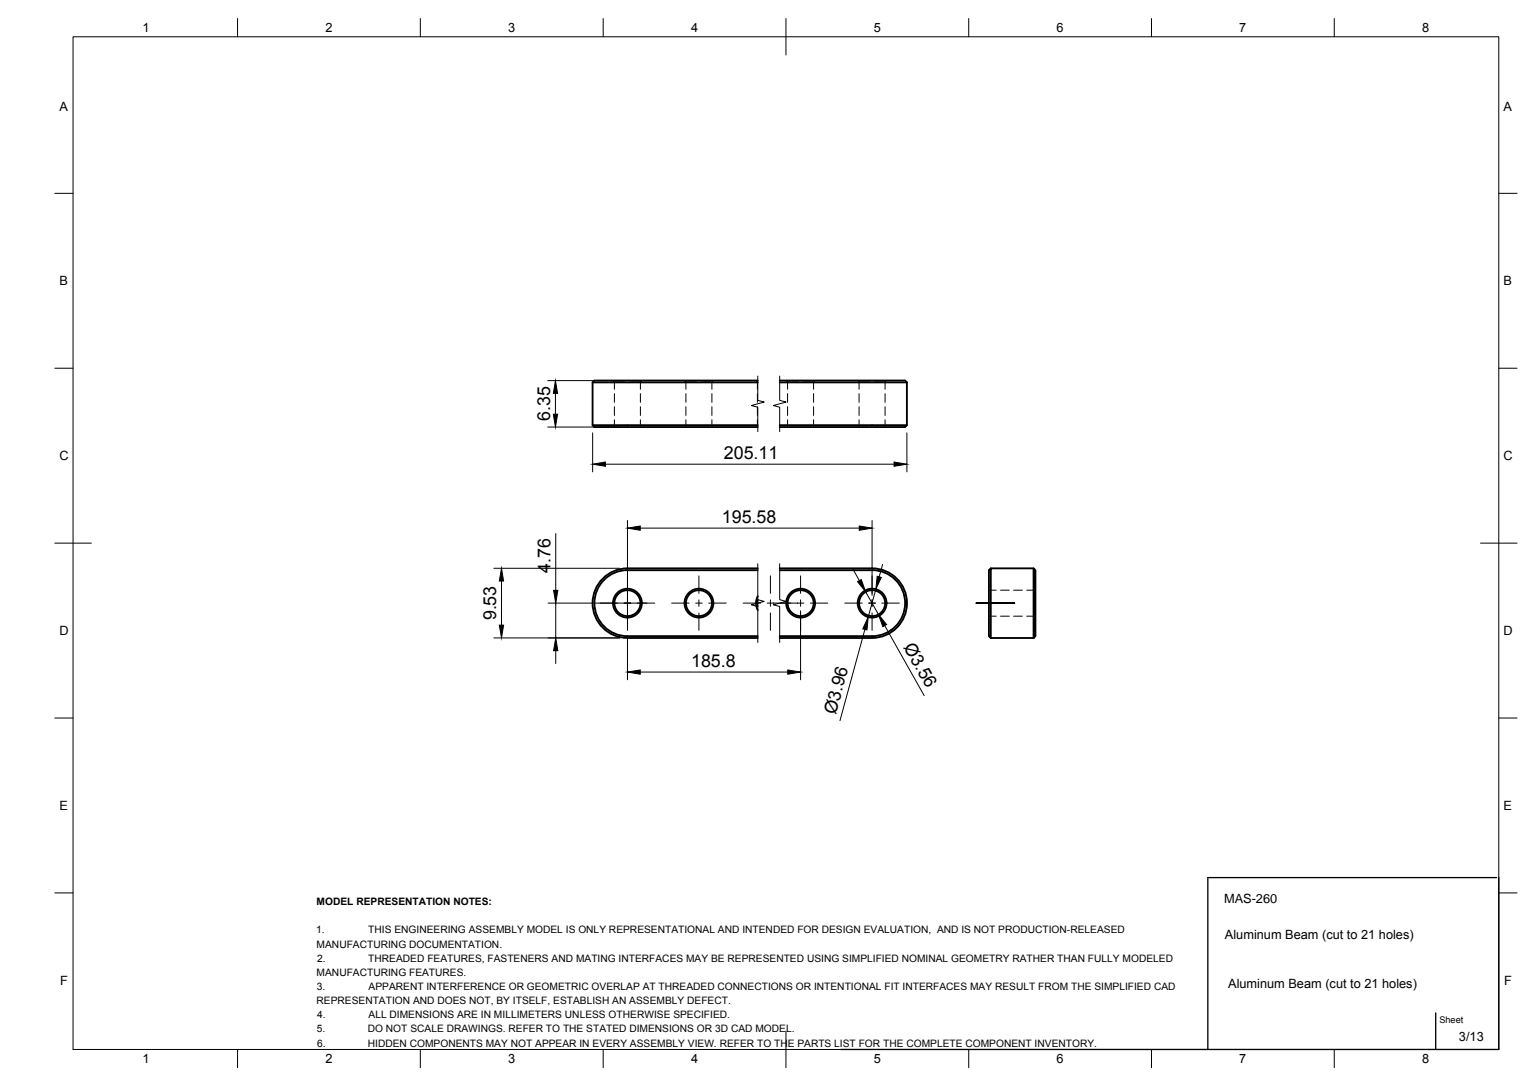
ISO-10303-21;
HEADER;
/* Generated by software containing ST-Developer
 * from STEP Tools, Inc. (www.steptools.com) 
 */

FILE_DESCRIPTION(
/* description */ (''),
/* implementation_level */ '2;1');

FILE_NAME(
/* name */ 'Aluminum Beam (cut to 21 holes).step',
/* time_stamp */ '2026-10-15T13:29:10-07:00',
/* author */ (''),
/* organization */ (''),
/* preprocessor_version */ 'ST-DEVELOPER v20.2',
/* originating_system */ 'Autodesk Translation Framework v15.15.0.0',
/* authorisation */ '');

FILE_SCHEMA (('AUTOMOTIVE_DESIGN { 1 0 10303 214 3 1 1 }'));
ENDSEC;

DATA;
#10=MECHANICAL_DESIGN_GEOMETRIC_PRESENTATION_REPRESENTATION('',(#938),#83219);
#910=SHAPE_REPRESENTATION_RELATIONSHIP('SRR','None',#83305,#924);
#924=ADVANCED_BREP_SHAPE_REPRESENTATION('',(#952),#83210);
#938=STYLED_ITEM('',(#83384),#952);
#952=MANIFOLD_SOLID_BREP('Body1',#26934);
#1019=FACE_BOUND('',#4280,.T.);
#1020=FACE_BOUND('',#4281,.T.);
#1021=FACE_BOUND('',#4282,.T.);
#1022=FACE_BOUND('',#4283,.T.);
#1023=FACE_BOUND('',#4284,.T.);
#1024=FACE_BOUND('',#4285,.T.);
#1025=FACE_BOUND('',#4286,.T.);
#1026=FACE_BOUND('',#4287,.T.);
#1027=FACE_BOUND('',#4288,.T.);
#1028=FACE_BOUND('',#4289,.T.);
#1029=FACE_BOUND('',#4290,.T.);
#1030=FACE_BOUND('',#4291,.T.);
#1031=FACE_BOUND('',#4292,.T.);
#1032=FACE_BOUND('',#4293,.T.);
#1033=FACE_BOUND('',#4294,.T.);
#1034=FACE_BOUND('',#4295,.T.);
#1035=FACE_BOUND('',#4296,.T.);
#1036=FACE_BOUND('',#4297,.T.);
#1037=FACE_BOUND('',#4298,.T.);
#1038=FACE_BOUND('',#4299,.T.);
#1039=FACE_BOUND('',#4300,.T.);
#1040=FACE_BOUND('',#4354,.T.);
#1041=FACE_BOUND('',#4355,.T.);
#1042=FACE_BOUND('',#4356,.T.);
#1043=FACE_BOUND('',#4357,.T.);
#1044=FACE_BOUND('',#4358,.T.);
#1045=FACE_BOUND('',#4359,.T.);
#1046=FACE_BOUND('',#4360,.T.);
#1047=FACE_BOUND('',#4361,.T.);
#1048=FACE_BOUND('',#4362,.T.);
#1049=FACE_BOUND('',#4363,.T.);
#1050=FACE_BOUND('',#4364,.T.);
#1051=FACE_BOUND('',#4365,.T.);
#1052=FACE_BOUND('',#4366,.T.);
#1053=FACE_BOUND('',#4367,.T.);
#1054=FACE_BOUND('',#4368,.T.);
#1055=FACE_BOUND('',#4369,.T.);
#1056=FACE_BOUND('',#4370,.T.);
#1057=FACE_BOUND('',#4371,.T.);
#1058=FACE_BOUND('',#4372,.T.);
#1059=FACE_BOUND('',#4373,.T.);
#1060=FACE_BOUND('',#4374,.T.);
#1415=PLANE('',#27876);
#1416=PLANE('',#27981);
#1417=PLANE('',#27984);
#1418=PLANE('',#27989);
#1419=PLANE('',#27990);
#1420=PLANE('',#27994);
#1421=PLANE('',#27998);
#1422=PLANE('',#27999);
#2259=CYLINDRICAL_SURFACE('',#27899,1.778);
#2260=CYLINDRICAL_SURFACE('',#27903,1.778);
#2261=CYLINDRICAL_SURFACE('',#27907,1.778);
#2262=CYLINDRICAL_SURFACE('',#27911,1.778);
#2263=CYLINDRICAL_SURFACE('',#27915,1.778);
#2264=CYLINDRICAL_SURFACE('',#27919,1.778);
#2265=CYLINDRICAL_SURFACE('',#27923,1.778);
#2266=CYLINDRICAL_SURFACE('',#27927,1.778);
#2267=CYLINDRICAL_SURFACE('',#27931,1.778);
#2268=CYLINDRICAL_SURFACE('',#27935,1.778);
#2269=CYLINDRICAL_SURFACE('',#27939,1.778);
#2270=CYLINDRICAL_SURFACE('',#27943,1.778);
#2271=CYLINDRICAL_SURFACE('',#27947,1.778);
#2272=CYLINDRICAL_SURFACE('',#27951,1.778);
#2273=CYLINDRICAL_SURFACE('',#27955,1.778);
#2274=CYLINDRICAL_SURFACE('',#27959,1.778);
#2275=CYLINDRICAL_SURFACE('',#27963,1.778);
#2276=CYLINDRICAL_SURFACE('',#27967,1.778);
#2277=CYLINDRICAL_SURFACE('',#27971,1.778);
#2278=CYLINDRICAL_SURFACE('',#27975,1.778);
#2279=CYLINDRICAL_SURFACE('',#27979,1.778);
#2280=CYLINDRICAL_SURFACE('',#27987,4.7625);
#2281=CYLINDRICAL_SURFACE('',#27997,4.7625);
#2841=FACE_OUTER_BOUND('',#4278,.T.);
#2842=FACE_OUTER_BOUND('',#4279,.T.);
#2843=FACE_OUTER_BOUND('',#4301,.T.);
#2844=FACE_OUTER_BOUND('',#4302,.T.);
#2845=FACE_OUTER_BOUND('',#4303,.T.);
#2846=FACE_OUTER_BOUND('',#4304,.T.);
#2847=FACE_OUTER_BOUND('',#4305,.T.);
#2848=FACE_OUTER_BOUND('',#4306,.T.);
#2849=FACE_OUTER_BOUND('',#4307,.T.);
#2850=FACE_OUTER_BOUND('',#4308,.T.);
#2851=FACE_OUTER_BOUND('',#4309,.T.);
#2852=FACE_OUTER_BOUND('',#4310,.T.);
#2853=FACE_OUTER_BOUND('',#4311,.T.);
#2854=FACE_OUTER_BOUND('',#4312,.T.);
#2855=FACE_OUTER_BOUND('',#4313,.T.);
#2856=FACE_OUTER_BOUND('',#4314,.T.);
#2857=FACE_OUTER_BOUND('',#4315,.T.);
#2858=FACE_OUTER_BOUND('',#4316,.T.);
#2859=FACE_OUTER_BOUND('',#4317,.T.);
#2860=FACE_OUTER_BOUND('',#4318,.T.);
#2861=FACE_OUTER_BOUND('',#4319,.T.);
#2862=FACE_OUTER_BOUND('',#4320,.T.);
#2863=FACE_OUTER_BOUND('',#4321,.T.);
#2864=FACE_OUTER_BOUND('',#4322,.T.);
#2865=FACE_OUTER_BOUND('',#4323,.T.);
#2866=FACE_OUTER_BOUND('',#4324,.T.);
#2867=FACE_OUTER_BOUND('',#4325,.T.);
#2868=FACE_OUTER_BOUND('',#4326,.T.);
#2869=FACE_OUTER_BOUND('',#4327,.T.);
#2870=FACE_OUTER_BOUND('',#4328,.T.);
#2871=FACE_OUTER_BOUND('',#4329,.T.);
#2872=FACE_OUTER_BOUND('',#4330,.T.);
#2873=FACE_OUTER_BOUND('',#4331,.T.);
#2874=FACE_OUTER_BOUND('',#4332,.T.);
#2875=FACE_OUTER_BOUND('',#4333,.T.);
#2876=FACE_OUTER_BOUND('',#4334,.T.);
#2877=FACE_OUTER_BOUND('',#4335,.T.);
#2878=FACE_OUTER_BOUND('',#4336,.T.);
#2879=FACE_OUTER_BOUND('',#4337,.T.);
#2880=FACE_OUTER_BOUND('',#4338,.T.);
#2881=FACE_OUTER_BOUND('',#4339,.T.);
#2882=FACE_OUTER_BOUND('',#4340,.T.);
#2883=FACE_OUTER_BOUND('',#4341,.T.);
#2884=FACE_OUTER_BOUND('',#4342,.T.);
#2885=FACE_OUTER_BOUND('',#4343,.T.);
#2886=FACE_OUTER_BOUND('',#4344,.T.);
#2887=FACE_OUTER_BOUND('',#4345,.T.);
#2888=FACE_OUTER_BOUND('',#4346,.T.);
#2889=FACE_OUTER_BOUND('',#4347,.T.);
#2890=FACE_OUTER_BOUND('',#4348,.T.);
#2891=FACE_OUTER_BOUND('',#4349,.T.);
#2892=FACE_OUTER_BOUND('',#4350,.T.);
#2893=FACE_OUTER_BOUND('',#4351,.T.);
#2894=FACE_OUTER_BOUND('',#4352,.T.);
#2895=FACE_OUTER_BOUND('',#4353,.T.);
#2896=FACE_OUTER_BOUND('',#4375,.T.);
#4278=EDGE_LOOP('',(#20208,#20209,#20210,#20211));
#4279=EDGE_LOOP('',(#20212,#20213,#20214,#20215));
#4280=EDGE_LOOP('',(#20216));
#4281=EDGE_LOOP('',(#20217));
#4282=EDGE_LOOP('',(#20218));
#4283=EDGE_LOOP('',(#20219));
#4284=EDGE_LOOP('',(#20220));
#4285=EDGE_LOOP('',(#20221));
#4286=EDGE_LOOP('',(#20222));
#4287=EDGE_LOOP('',(#20223));
#4288=EDGE_LOOP('',(#20224));
#4289=EDGE_LOOP('',(#20225));
#4290=EDGE_LOOP('',(#20226));
#4291=EDGE_LOOP('',(#20227));
#4292=EDGE_LOOP('',(#20228));
#4293=EDGE_LOOP('',(#20229));
#4294=EDGE_LOOP('',(#20230));
#4295=EDGE_LOOP('',(#20231));
#4296=EDGE_LOOP('',(#20232));
#4297=EDGE_LOOP('',(#20233));
#4298=EDGE_LOOP('',(#20234));
#4299=EDGE_LOOP('',(#20235));
#4300=EDGE_LOOP('',(#20236));
#4301=EDGE_LOOP('',(#20237,#20238,#20239,#20240));
#4302=EDGE_LOOP('',(#20241,#20242,#20243,#20244));
#4303=EDGE_LOOP('',(#20245,#20246,#20247,#20248));
#4304=EDGE_LOOP('',(#20249,#20250,#20251,#20252));
#4305=EDGE_LOOP('',(#20253,#20254,#20255,#20256));
#4306=EDGE_LOOP('',(#20257,#20258,#20259,#20260));
#4307=EDGE_LOOP('',(#20261,#20262,#20263,#20264));
#4308=EDGE_LOOP('',(#20265,#20266,#20267,#20268));
#4309=EDGE_LOOP('',(#20269,#20270,#20271,#20272));
#4310=EDGE_LOOP('',(#20273,#20274,#20275,#20276));
#4311=EDGE_LOOP('',(#20277,#20278,#20279,#20280));
#4312=EDGE_LOOP('',(#20281,#20282,#20283,#20284));
#4313=EDGE_LOOP('',(#20285,#20286,#20287,#20288));
#4314=EDGE_LOOP('',(#20289,#20290,#20291,#20292));
#4315=EDGE_LOOP('',(#20293,#20294,#20295,#20296));
#4316=EDGE_LOOP('',(#20297,#20298,#20299,#20300));
#4317=EDGE_LOOP('',(#20301,#20302,#20303,#20304));
#4318=EDGE_LOOP('',(#20305,#20306,#20307,#20308));
#4319=EDGE_LOOP('',(#20309,#20310,#20311,#20312));
#4320=EDGE_LOOP('',(#20313,#20314,#20315,#20316));
#4321=EDGE_LOOP('',(#20317,#20318,#20319,#20320));
#4322=EDGE_LOOP('',(#20321,#20322,#20323,#20324));
#4323=EDGE_LOOP('',(#20325,#20326,#20327,#20328));
#4324=EDGE_LOOP('',(#20329,#20330,#20331,#20332));
#4325=EDGE_LOOP('',(#20333,#20334,#20335,#20336));
#4326=EDGE_LOOP('',(#20337,#20338,#20339,#20340));
#4327=EDGE_LOOP('',(#20341,#20342,#20343,#20344));
#4328=EDGE_LOOP('',(#20345,#20346,#20347,#20348));
#4329=EDGE_LOOP('',(#20349,#20350,#20351,#20352));
#4330=EDGE_LOOP('',(#20353,#20354,#20355,#20356));
#4331=EDGE_LOOP('',(#20357,#20358,#20359,#20360));
#4332=EDGE_LOOP('',(#20361,#20362,#20363,#20364));
#4333=EDGE_LOOP('',(#20365,#20366,#20367,#20368));
#4334=EDGE_LOOP('',(#20369,#20370,#20371,#20372));
#4335=EDGE_LOOP('',(#20373,#20374,#20375,#20376));
#4336=EDGE_LOOP('',(#20377,#20378,#20379,#20380));
#4337=EDGE_LOOP('',(#20381,#20382,#20383,#20384));
#4338=EDGE_LOOP('',(#20385,#20386,#20387,#20388));
#4339=EDGE_LOOP('',(#20389,#20390,#20391,#20392));
#4340=EDGE_LOOP('',(#20393,#20394,#20395,#20396));
#4341=EDGE_LOOP('',(#20397,#20398,#20399,#20400));
#4342=EDGE_LOOP('',(#20401,#20402,#20403,#20404));
#4343=EDGE_LOOP('',(#20405,#20406,#20407,#20408));
#4344=EDGE_LOOP('',(#20409,#20410,#20411,#20412));
#4345=EDGE_LOOP('',(#20413,#20414,#20415,#20416));
#4346=EDGE_LOOP('',(#20417,#20418,#20419,#20420));
#4347=EDGE_LOOP('',(#20421,#20422,#20423,#20424));
#4348=EDGE_LOOP('',(#20425,#20426,#20427,#20428));
#4349=EDGE_LOOP('',(#20429,#20430,#20431,#20432));
#4350=EDGE_LOOP('',(#20433,#20434,#20435,#20436));
#4351=EDGE_LOOP('',(#20437,#20438,#20439,#20440));
#4352=EDGE_LOOP('',(#20441,#20442,#20443,#20444));
#4353=EDGE_LOOP('',(#20445,#20446,#20447,#20448));
#4354=EDGE_LOOP('',(#20449));
#4355=EDGE_LOOP('',(#20450));
#4356=EDGE_LOOP('',(#20451));
#4357=EDGE_LOOP('',(#20452));
#4358=EDGE_LOOP('',(#20453));
#4359=EDGE_LOOP('',(#20454));
#4360=EDGE_LOOP('',(#20455));
#4361=EDGE_LOOP('',(#20456));
#4362=EDGE_LOOP('',(#20457));
#4363=EDGE_LOOP('',(#20458));
#4364=EDGE_LOOP('',(#20459));
#4365=EDGE_LOOP('',(#20460));
#4366=EDGE_LOOP('',(#20461));
#4367=EDGE_LOOP('',(#20462));
#4368=EDGE_LOOP('',(#20463));
#4369=EDGE_LOOP('',(#20464));
#4370=EDGE_LOOP('',(#20465));
#4371=EDGE_LOOP('',(#20466));
#4372=EDGE_LOOP('',(#20467));
#4373=EDGE_LOOP('',(#20468));
#4374=EDGE_LOOP('',(#20469));
#4375=EDGE_LOOP('',(#20470,#20471,#20472,#20473));
#6053=LINE('',#50676,#8564);
#6054=LINE('',#50681,#8565);
#6055=LINE('',#50685,#8566);
#6056=LINE('',#50729,#8567);
#6057=LINE('',#50734,#8568);
#6058=LINE('',#50737,#8569);
#6059=LINE('',#50742,#8570);
#6060=LINE('',#50745,#8571);
#6061=LINE('',#50750,#8572);
#6062=LINE('',#50753,#8573);
#6063=LINE('',#50758,#8574);
#6064=LINE('',#50761,#8575);
#6065=LINE('',#50766,#8576);
#6066=LINE('',#50769,#8577);
#6067=LINE('',#50774,#8578);
#6068=LINE('',#50777,#8579);
#6069=LINE('',#50782,#8580);
#6070=LINE('',#50785,#8581);
#6071=LINE('',#50790,#8582);
#6072=LINE('',#50793,#8583);
#6073=LINE('',#50798,#8584);
#6074=LINE('',#50801,#8585);
#6075=LINE('',#50806,#8586);
#6076=LINE('',#50809,#8587);
#6077=LINE('',#50814,#8588);
#6078=LINE('',#50817,#8589);
#6079=LINE('',#50822,#8590);
#6080=LINE('',#50825,#8591);
#6081=LINE('',#50830,#8592);
#6082=LINE('',#50833,#8593);
#6083=LINE('',#50838,#8594);
#6084=LINE('',#50841,#8595);
#6085=LINE('',#50846,#8596);
#6086=LINE('',#50849,#8597);
#6087=LINE('',#50854,#8598);
#6088=LINE('',#50857,#8599);
#6089=LINE('',#50862,#8600);
#6090=LINE('',#50865,#8601);
#6091=LINE('',#50870,#8602);
#6092=LINE('',#50873,#8603);
#6093=LINE('',#50878,#8604);
#6094=LINE('',#50881,#8605);
#6095=LINE('',#50886,#8606);
#6096=LINE('',#50889,#8607);
#6097=LINE('',#50893,#8608);
#6098=LINE('',#50895,#8609);
#6099=LINE('',#50896,#8610);
#6100=LINE('',#50899,#8611);
#6101=LINE('',#50903,#8612);
#6102=LINE('',#50904,#8613);
#6103=LINE('',#50909,#8614);
#6104=LINE('',#50912,#8615);
#6105=LINE('',#50915,#8616);
#6106=LINE('',#50916,#8617);
#6107=LINE('',#50919,#8618);
#6108=LINE('',#50921,#8619);
#6109=LINE('',#50922,#8620);
#6110=LINE('',#50927,#8621);
#6111=LINE('',#50931,#8622);
#6112=LINE('',#50932,#8623);
#6113=LINE('',#50933,#8624);
#6114=LINE('',#50937,#8625);
#8564=VECTOR('',#31585,1.87799999999999);
#8565=VECTOR('',#31590,10.);
#8566=VECTOR('',#31593,10.);
#8567=VECTOR('',#31638,1.778);
#8568=VECTOR('',#31645,1.87799999999999);
#8569=VECTOR('',#31648,1.778);
#8570=VECTOR('',#31655,1.878);
#8571=VECTOR('',#31658,1.778);
#8572=VECTOR('',#31665,1.878);
#8573=VECTOR('',#31668,1.778);
#8574=VECTOR('',#31675,1.878);
#8575=VECTOR('',#31678,1.778);
#8576=VECTOR('',#31685,1.87799999999999);
#8577=VECTOR('',#31688,1.778);
#8578=VECTOR('',#31695,1.878);
#8579=VECTOR('',#31698,1.778);
#8580=VECTOR('',#31705,1.878);
#8581=VECTOR('',#31708,1.778);
#8582=VECTOR('',#31715,1.878);
#8583=VECTOR('',#31718,1.778);
#8584=VECTOR('',#31725,1.878);
#8585=VECTOR('',#31728,1.778);
#8586=VECTOR('',#31735,1.87799999999999);
#8587=VECTOR('',#31738,1.778);
#8588=VECTOR('',#31745,1.878);
#8589=VECTOR('',#31748,1.778);
#8590=VECTOR('',#31755,1.878);
#8591=VECTOR('',#31758,1.778);
#8592=VECTOR('',#31765,1.878);
#8593=VECTOR('',#31768,1.778);
#8594=VECTOR('',#31775,1.878);
#8595=VECTOR('',#31778,1.778);
#8596=VECTOR('',#31785,1.878);
#8597=VECTOR('',#31788,1.778);
#8598=VECTOR('',#31795,1.878);
#8599=VECTOR('',#31798,1.778);
#8600=VECTOR('',#31805,1.878);
#8601=VECTOR('',#31808,1.778);
#8602=VECTOR('',#31815,1.878);
#8603=VECTOR('',#31818,1.778);
#8604=VECTOR('',#31825,1.878);
#8605=VECTOR('',#31828,1.778);
#8606=VECTOR('',#31835,1.87799999999999);
#8607=VECTOR('',#31838,1.778);
#8608=VECTOR('',#31843,10.);
#8609=VECTOR('',#31844,10.);
#8610=VECTOR('',#31845,10.);
#8611=VECTOR('',#31848,9.99999999999999);
#8612=VECTOR('',#31853,10.);
#8613=VECTOR('',#31854,10.);
#8614=VECTOR('',#31861,10.);
#8615=VECTOR('',#31864,10.);
#8616=VECTOR('',#31867,10.);
#8617=VECTOR('',#31868,10.);
#8618=VECTOR('',#31871,10.);
#8619=VECTOR('',#31872,10.);
#8620=VECTOR('',#31873,10.);
#8621=VECTOR('',#31878,9.99999999999999);
#8622=VECTOR('',#31883,10.);
#8623=VECTOR('',#31884,10.);
#8624=VECTOR('',#31885,10.);
#8625=VECTOR('',#31892,10.);
#10617=CIRCLE('',#27874,1.778);
#10618=CIRCLE('',#27875,1.97799999999999);
#10619=CIRCLE('',#27877,4.51249999999999);
#10620=CIRCLE('',#27878,4.5125);
#10621=CIRCLE('',#27879,1.97799999999999);
#10622=CIRCLE('',#27880,1.978);
#10623=CIRCLE('',#27881,1.97799999999999);
#10624=CIRCLE('',#27882,1.978);
#10625=CIRCLE('',#27883,1.978);
#10626=CIRCLE('',#27884,1.978);
#10627=CIRCLE('',#27885,1.978);
#10628=CIRCLE('',#27886,1.978);
#10629=CIRCLE('',#27887,1.978);
#10630=CIRCLE('',#27888,1.978);
#10631=CIRCLE('',#27889,1.97799999999999);
#10632=CIRCLE('',#27890,1.978);
#10633=CIRCLE('',#27891,1.978);
#10634=CIRCLE('',#27892,1.978);
#10635=CIRCLE('',#27893,1.978);
#10636=CIRCLE('',#27894,1.97799999999999);
#10637=CIRCLE('',#27895,1.978);
#10638=CIRCLE('',#27896,1.978);
#10639=CIRCLE('',#27897,1.978);
#10640=CIRCLE('',#27898,1.978);
#10641=CIRCLE('',#27900,1.778);
#10642=CIRCLE('',#27902,1.778);
#10643=CIRCLE('',#27904,1.778);
#10644=CIRCLE('',#27906,1.778);
#10645=CIRCLE('',#27908,1.778);
#10646=CIRCLE('',#27910,1.778);
#10647=CIRCLE('',#27912,1.778);
#10648=CIRCLE('',#27914,1.778);
#10649=CIRCLE('',#27916,1.778);
#10650=CIRCLE('',#27918,1.778);
#10651=CIRCLE('',#27920,1.778);
#10652=CIRCLE('',#27922,1.778);
#10653=CIRCLE('',#27924,1.778);
#10654=CIRCLE('',#27926,1.778);
#10655=CIRCLE('',#27928,1.778);
#10656=CIRCLE('',#27930,1.778);
#10657=CIRCLE('',#27932,1.778);
#10658=CIRCLE('',#27934,1.778);
#10659=CIRCLE('',#27936,1.778);
#10660=CIRCLE('',#27938,1.778);
#10661=CIRCLE('',#27940,1.778);
#10662=CIRCLE('',#27942,1.778);
#10663=CIRCLE('',#27944,1.778);
#10664=CIRCLE('',#27946,1.778);
#10665=CIRCLE('',#27948,1.778);
#10666=CIRCLE('',#27950,1.778);
#10667=CIRCLE('',#27952,1.778);
#10668=CIRCLE('',#27954,1.778);
#10669=CIRCLE('',#27956,1.778);
#10670=CIRCLE('',#27958,1.778);
#10671=CIRCLE('',#27960,1.778);
#10672=CIRCLE('',#27962,1.778);
#10673=CIRCLE('',#27964,1.778);
#10674=CIRCLE('',#27966,1.778);
#10675=CIRCLE('',#27968,1.778);
#10676=CIRCLE('',#27970,1.778);
#10677=CIRCLE('',#27972,1.778);
#10678=CIRCLE('',#27974,1.778);
#10679=CIRCLE('',#27976,1.778);
#10680=CIRCLE('',#27978,1.778);
#10681=CIRCLE('',#27980,1.778);
#10682=CIRCLE('',#27983,4.7625);
#10683=CIRCLE('',#27986,4.7625);
#10684=CIRCLE('',#27988,4.7625);
#10685=CIRCLE('',#27992,4.7625);
#10686=CIRCLE('',#27993,4.5125);
#10687=CIRCLE('',#27996,4.51249999999999);
#11900=VERTEX_POINT('',#50673);
#11901=VERTEX_POINT('',#50675);
#11902=VERTEX_POINT('',#50679);
#11903=VERTEX_POINT('',#50680);
#11904=VERTEX_POINT('',#50682);
#11905=VERTEX_POINT('',#50684);
#11906=VERTEX_POINT('',#50687);
#11907=VERTEX_POINT('',#50689);
#11908=VERTEX_POINT('',#50691);
#11909=VERTEX_POINT('',#50693);
#11910=VERTEX_POINT('',#50695);
#11911=VERTEX_POINT('',#50697);
#11912=VERTEX_POINT('',#50699);
#11913=VERTEX_POINT('',#50701);
#11914=VERTEX_POINT('',#50703);
#11915=VERTEX_POINT('',#50705);
#11916=VERTEX_POINT('',#50707);
#11917=VERTEX_POINT('',#50709);
#11918=VERTEX_POINT('',#50711);
#11919=VERTEX_POINT('',#50713);
#11920=VERTEX_POINT('',#50715);
#11921=VERTEX_POINT('',#50717);
#11922=VERTEX_POINT('',#50719);
#11923=VERTEX_POINT('',#50721);
#11924=VERTEX_POINT('',#50723);
#11925=VERTEX_POINT('',#50725);
#11926=VERTEX_POINT('',#50728);
#11927=VERTEX_POINT('',#50732);
#11928=VERTEX_POINT('',#50736);
#11929=VERTEX_POINT('',#50740);
#11930=VERTEX_POINT('',#50744);
#11931=VERTEX_POINT('',#50748);
#11932=VERTEX_POINT('',#50752);
#11933=VERTEX_POINT('',#50756);
#11934=VERTEX_POINT('',#50760);
#11935=VERTEX_POINT('',#50764);
#11936=VERTEX_POINT('',#50768);
#11937=VERTEX_POINT('',#50772);
#11938=VERTEX_POINT('',#50776);
#11939=VERTEX_POINT('',#50780);
#11940=VERTEX_POINT('',#50784);
#11941=VERTEX_POINT('',#50788);
#11942=VERTEX_POINT('',#50792);
#11943=VERTEX_POINT('',#50796);
#11944=VERTEX_POINT('',#50800);
#11945=VERTEX_POINT('',#50804);
#11946=VERTEX_POINT('',#50808);
#11947=VERTEX_POINT('',#50812);
#11948=VERTEX_POINT('',#50816);
#11949=VERTEX_POINT('',#50820);
#11950=VERTEX_POINT('',#50824);
#11951=VERTEX_POINT('',#50828);
#11952=VERTEX_POINT('',#50832);
#11953=VERTEX_POINT('',#50836);
#11954=VERTEX_POINT('',#50840);
#11955=VERTEX_POINT('',#50844);
#11956=VERTEX_POINT('',#50848);
#11957=VERTEX_POINT('',#50852);
#11958=VERTEX_POINT('',#50856);
#11959=VERTEX_POINT('',#50860);
#11960=VERTEX_POINT('',#50864);
#11961=VERTEX_POINT('',#50868);
#11962=VERTEX_POINT('',#50872);
#11963=VERTEX_POINT('',#50876);
#11964=VERTEX_POINT('',#50880);
#11965=VERTEX_POINT('',#50884);
#11966=VERTEX_POINT('',#50888);
#11967=VERTEX_POINT('',#50892);
#11968=VERTEX_POINT('',#50894);
#11969=VERTEX_POINT('',#50898);
#11970=VERTEX_POINT('',#50902);
#11971=VERTEX_POINT('',#50908);
#11972=VERTEX_POINT('',#50910);
#11973=VERTEX_POINT('',#50914);
#11974=VERTEX_POINT('',#50918);
#11975=VERTEX_POINT('',#50920);
#11976=VERTEX_POINT('',#50924);
#11977=VERTEX_POINT('',#50926);
#11978=VERTEX_POINT('',#50930);
#14965=EDGE_CURVE('',#11900,#11900,#10617,.T.);
#14966=EDGE_CURVE('',#11900,#11901,#6053,.T.);
#14967=EDGE_CURVE('',#11901,#11901,#10618,.T.);
#14968=EDGE_CURVE('',#11902,#11903,#6054,.T.);
#14969=EDGE_CURVE('',#11904,#11902,#10619,.T.);
#14970=EDGE_CURVE('',#11905,#11904,#6055,.T.);
#14971=EDGE_CURVE('',#11903,#11905,#10620,.T.);
#14972=EDGE_CURVE('',#11906,#11906,#10621,.T.);
#14973=EDGE_CURVE('',#11907,#11907,#10622,.T.);
#14974=EDGE_CURVE('',#11908,#11908,#10623,.T.);
#14975=EDGE_CURVE('',#11909,#11909,#10624,.T.);
#14976=EDGE_CURVE('',#11910,#11910,#10625,.T.);
#14977=EDGE_CURVE('',#11911,#11911,#10626,.T.);
#14978=EDGE_CURVE('',#11912,#11912,#10627,.T.);
#14979=EDGE_CURVE('',#11913,#11913,#10628,.T.);
#14980=EDGE_CURVE('',#11914,#11914,#10629,.T.);
#14981=EDGE_CURVE('',#11915,#11915,#10630,.T.);
#14982=EDGE_CURVE('',#11916,#11916,#10631,.T.);
#14983=EDGE_CURVE('',#11917,#11917,#10632,.T.);
#14984=EDGE_CURVE('',#11918,#11918,#10633,.T.);
#14985=EDGE_CURVE('',#11919,#11919,#10634,.T.);
#14986=EDGE_CURVE('',#11920,#11920,#10635,.T.);
#14987=EDGE_CURVE('',#11921,#11921,#10636,.T.);
#14988=EDGE_CURVE('',#11922,#11922,#10637,.T.);
#14989=EDGE_CURVE('',#11923,#11923,#10638,.T.);
#14990=EDGE_CURVE('',#11924,#11924,#10639,.T.);
#14991=EDGE_CURVE('',#11925,#11925,#10640,.T.);
#14992=EDGE_CURVE('',#11900,#11926,#6056,.T.);
#14993=EDGE_CURVE('',#11926,#11926,#10641,.T.);
#14994=EDGE_CURVE('',#11927,#11927,#10642,.T.);
#14995=EDGE_CURVE('',#11927,#11906,#6057,.T.);
#14996=EDGE_CURVE('',#11927,#11928,#6058,.T.);
#14997=EDGE_CURVE('',#11928,#11928,#10643,.T.);
#14998=EDGE_CURVE('',#11929,#11929,#10644,.T.);
#14999=EDGE_CURVE('',#11929,#11925,#6059,.T.);
#15000=EDGE_CURVE('',#11929,#11930,#6060,.T.);
#15001=EDGE_CURVE('',#11930,#11930,#10645,.T.);
#15002=EDGE_CURVE('',#11931,#11931,#10646,.T.);
#15003=EDGE_CURVE('',#11931,#11907,#6061,.T.);
#15004=EDGE_CURVE('',#11931,#11932,#6062,.T.);
#15005=EDGE_CURVE('',#11932,#11932,#10647,.T.);
#15006=EDGE_CURVE('',#11933,#11933,#10648,.T.);
#15007=EDGE_CURVE('',#11933,#11924,#6063,.T.);
#15008=EDGE_CURVE('',#11933,#11934,#6064,.T.);
#15009=EDGE_CURVE('',#11934,#11934,#10649,.T.);
#15010=EDGE_CURVE('',#11935,#11935,#10650,.T.);
#15011=EDGE_CURVE('',#11935,#11908,#6065,.T.);
#15012=EDGE_CURVE('',#11935,#11936,#6066,.T.);
#15013=EDGE_CURVE('',#11936,#11936,#10651,.T.);
#15014=EDGE_CURVE('',#11937,#11937,#10652,.T.);
#15015=EDGE_CURVE('',#11937,#11923,#6067,.T.);
#15016=EDGE_CURVE('',#11937,#11938,#6068,.T.);
#15017=EDGE_CURVE('',#11938,#11938,#10653,.T.);
#15018=EDGE_CURVE('',#11939,#11939,#10654,.T.);
#15019=EDGE_CURVE('',#11939,#11909,#6069,.T.);
#15020=EDGE_CURVE('',#11939,#11940,#6070,.T.);
#15021=EDGE_CURVE('',#11940,#11940,#10655,.T.);
#15022=EDGE_CURVE('',#11941,#11941,#10656,.T.);
#15023=EDGE_CURVE('',#11941,#11922,#6071,.T.);
#15024=EDGE_CURVE('',#11941,#11942,#6072,.T.);
#15025=EDGE_CURVE('',#11942,#11942,#10657,.T.);
#15026=EDGE_CURVE('',#11943,#11943,#10658,.T.);
#15027=EDGE_CURVE('',#11943,#11910,#6073,.T.);
#15028=EDGE_CURVE('',#11943,#11944,#6074,.T.);
#15029=EDGE_CURVE('',#11944,#11944,#10659,.T.);
#15030=EDGE_CURVE('',#11945,#11945,#10660,.T.);
#15031=EDGE_CURVE('',#11945,#11921,#6075,.T.);
#15032=EDGE_CURVE('',#11945,#11946,#6076,.T.);
#15033=EDGE_CURVE('',#11946,#11946,#10661,.T.);
#15034=EDGE_CURVE('',#11947,#11947,#10662,.T.);
#15035=EDGE_CURVE('',#11947,#11911,#6077,.T.);
#15036=EDGE_CURVE('',#11947,#11948,#6078,.T.);
#15037=EDGE_CURVE('',#11948,#11948,#10663,.T.);
#15038=EDGE_CURVE('',#11949,#11949,#10664,.T.);
#15039=EDGE_CURVE('',#11949,#11920,#6079,.T.);
#15040=EDGE_CURVE('',#11949,#11950,#6080,.T.);
#15041=EDGE_CURVE('',#11950,#11950,#10665,.T.);
#15042=EDGE_CURVE('',#11951,#11951,#10666,.T.);
#15043=EDGE_CURVE('',#11951,#11912,#6081,.T.);
#15044=EDGE_CURVE('',#11951,#11952,#6082,.T.);
#15045=EDGE_CURVE('',#11952,#11952,#10667,.T.);
#15046=EDGE_CURVE('',#11953,#11953,#10668,.T.);
#15047=EDGE_CURVE('',#11953,#11919,#6083,.T.);
#15048=EDGE_CURVE('',#11953,#11954,#6084,.T.);
#15049=EDGE_CURVE('',#11954,#11954,#10669,.T.);
#15050=EDGE_CURVE('',#11955,#11955,#10670,.T.);
#15051=EDGE_CURVE('',#11955,#11913,#6085,.T.);
#15052=EDGE_CURVE('',#11955,#11956,#6086,.T.);
#15053=EDGE_CURVE('',#11956,#11956,#10671,.T.);
#15054=EDGE_CURVE('',#11957,#11957,#10672,.T.);
#15055=EDGE_CURVE('',#11957,#11918,#6087,.T.);
#15056=EDGE_CURVE('',#11957,#11958,#6088,.T.);
#15057=EDGE_CURVE('',#11958,#11958,#10673,.T.);
#15058=EDGE_CURVE('',#11959,#11959,#10674,.T.);
#15059=EDGE_CURVE('',#11959,#11914,#6089,.T.);
#15060=EDGE_CURVE('',#11959,#11960,#6090,.T.);
#15061=EDGE_CURVE('',#11960,#11960,#10675,.T.);
#15062=EDGE_CURVE('',#11961,#11961,#10676,.T.);
#15063=EDGE_CURVE('',#11961,#11917,#6091,.T.);
#15064=EDGE_CURVE('',#11961,#11962,#6092,.T.);
#15065=EDGE_CURVE('',#11962,#11962,#10677,.T.);
#15066=EDGE_CURVE('',#11963,#11963,#10678,.T.);
#15067=EDGE_CURVE('',#11963,#11915,#6093,.T.);
#15068=EDGE_CURVE('',#11963,#11964,#6094,.T.);
#15069=EDGE_CURVE('',#11964,#11964,#10679,.T.);
#15070=EDGE_CURVE('',#11965,#11965,#10680,.T.);
#15071=EDGE_CURVE('',#11965,#11916,#6095,.T.);
#15072=EDGE_CURVE('',#11965,#11966,#6096,.T.);
#15073=EDGE_CURVE('',#11966,#11966,#10681,.T.);
#15074=EDGE_CURVE('',#11967,#11902,#6097,.T.);
#15075=EDGE_CURVE('',#11903,#11968,#6098,.T.);
#15076=EDGE_CURVE('',#11968,#11967,#6099,.T.);
#15077=EDGE_CURVE('',#11969,#11904,#6100,.T.);
#15078=EDGE_CURVE('',#11967,#11969,#10682,.T.);
#15079=EDGE_CURVE('',#11970,#11905,#6101,.T.);
#15080=EDGE_CURVE('',#11969,#11970,#6102,.T.);
#15081=EDGE_CURVE('',#11970,#11968,#10683,.T.);
#15082=EDGE_CURVE('',#11971,#11967,#6103,.T.);
#15083=EDGE_CURVE('',#11972,#11971,#10684,.T.);
#15084=EDGE_CURVE('',#11972,#11969,#6104,.T.);
#15085=EDGE_CURVE('',#11973,#11968,#6105,.T.);
#15086=EDGE_CURVE('',#11971,#11973,#6106,.T.);
#15087=EDGE_CURVE('',#11973,#11974,#6107,.T.);
#15088=EDGE_CURVE('',#11974,#11975,#6108,.T.);
#15089=EDGE_CURVE('',#11975,#11971,#6109,.T.);
#15090=EDGE_CURVE('',#11973,#11976,#10685,.T.);
#15091=EDGE_CURVE('',#11976,#11977,#6110,.T.);
#15092=EDGE_CURVE('',#11977,#11974,#10686,.T.);
#15093=EDGE_CURVE('',#11972,#11978,#6111,.T.);
#15094=EDGE_CURVE('',#11978,#11977,#6112,.T.);
#15095=EDGE_CURVE('',#11976,#11972,#6113,.T.);
#15096=EDGE_CURVE('',#11975,#11978,#10687,.T.);
#15097=EDGE_CURVE('',#11976,#11970,#6114,.T.);
#20208=ORIENTED_EDGE('',*,*,#14965,.T.);
#20209=ORIENTED_EDGE('',*,*,#14966,.T.);
#20210=ORIENTED_EDGE('',*,*,#14967,.T.);
#20211=ORIENTED_EDGE('',*,*,#14966,.F.);
#20212=ORIENTED_EDGE('',*,*,#14968,.F.);
#20213=ORIENTED_EDGE('',*,*,#14969,.F.);
#20214=ORIENTED_EDGE('',*,*,#14970,.F.);
#20215=ORIENTED_EDGE('',*,*,#14971,.F.);
#20216=ORIENTED_EDGE('',*,*,#14972,.F.);
#20217=ORIENTED_EDGE('',*,*,#14973,.F.);
#20218=ORIENTED_EDGE('',*,*,#14974,.F.);
#20219=ORIENTED_EDGE('',*,*,#14975,.F.);
#20220=ORIENTED_EDGE('',*,*,#14976,.F.);
#20221=ORIENTED_EDGE('',*,*,#14977,.F.);
#20222=ORIENTED_EDGE('',*,*,#14978,.F.);
#20223=ORIENTED_EDGE('',*,*,#14979,.F.);
#20224=ORIENTED_EDGE('',*,*,#14980,.F.);
#20225=ORIENTED_EDGE('',*,*,#14981,.F.);
#20226=ORIENTED_EDGE('',*,*,#14982,.F.);
#20227=ORIENTED_EDGE('',*,*,#14983,.F.);
#20228=ORIENTED_EDGE('',*,*,#14984,.F.);
#20229=ORIENTED_EDGE('',*,*,#14985,.F.);
#20230=ORIENTED_EDGE('',*,*,#14986,.F.);
#20231=ORIENTED_EDGE('',*,*,#14987,.F.);
#20232=ORIENTED_EDGE('',*,*,#14988,.F.);
#20233=ORIENTED_EDGE('',*,*,#14989,.F.);
#20234=ORIENTED_EDGE('',*,*,#14990,.F.);
#20235=ORIENTED_EDGE('',*,*,#14991,.F.);
#20236=ORIENTED_EDGE('',*,*,#14967,.F.);
#20237=ORIENTED_EDGE('',*,*,#14965,.F.);
#20238=ORIENTED_EDGE('',*,*,#14992,.T.);
#20239=ORIENTED_EDGE('',*,*,#14993,.F.);
#20240=ORIENTED_EDGE('',*,*,#14992,.F.);
#20241=ORIENTED_EDGE('',*,*,#14994,.T.);
#20242=ORIENTED_EDGE('',*,*,#14995,.T.);
#20243=ORIENTED_EDGE('',*,*,#14972,.T.);
#20244=ORIENTED_EDGE('',*,*,#14995,.F.);
#20245=ORIENTED_EDGE('',*,*,#14994,.F.);
#20246=ORIENTED_EDGE('',*,*,#14996,.T.);
#20247=ORIENTED_EDGE('',*,*,#14997,.F.);
#20248=ORIENTED_EDGE('',*,*,#14996,.F.);
#20249=ORIENTED_EDGE('',*,*,#14998,.T.);
#20250=ORIENTED_EDGE('',*,*,#14999,.T.);
#20251=ORIENTED_EDGE('',*,*,#14991,.T.);
#20252=ORIENTED_EDGE('',*,*,#14999,.F.);
#20253=ORIENTED_EDGE('',*,*,#14998,.F.);
#20254=ORIENTED_EDGE('',*,*,#15000,.T.);
#20255=ORIENTED_EDGE('',*,*,#15001,.F.);
#20256=ORIENTED_EDGE('',*,*,#15000,.F.);
#20257=ORIENTED_EDGE('',*,*,#15002,.T.);
#20258=ORIENTED_EDGE('',*,*,#15003,.T.);
#20259=ORIENTED_EDGE('',*,*,#14973,.T.);
#20260=ORIENTED_EDGE('',*,*,#15003,.F.);
#20261=ORIENTED_EDGE('',*,*,#15002,.F.);
#20262=ORIENTED_EDGE('',*,*,#15004,.T.);
#20263=ORIENTED_EDGE('',*,*,#15005,.F.);
#20264=ORIENTED_EDGE('',*,*,#15004,.F.);
#20265=ORIENTED_EDGE('',*,*,#15006,.T.);
#20266=ORIENTED_EDGE('',*,*,#15007,.T.);
#20267=ORIENTED_EDGE('',*,*,#14990,.T.);
#20268=ORIENTED_EDGE('',*,*,#15007,.F.);
#20269=ORIENTED_EDGE('',*,*,#15006,.F.);
#20270=ORIENTED_EDGE('',*,*,#15008,.T.);
#20271=ORIENTED_EDGE('',*,*,#15009,.F.);
#20272=ORIENTED_EDGE('',*,*,#15008,.F.);
#20273=ORIENTED_EDGE('',*,*,#15010,.T.);
#20274=ORIENTED_EDGE('',*,*,#15011,.T.);
#20275=ORIENTED_EDGE('',*,*,#14974,.T.);
#20276=ORIENTED_EDGE('',*,*,#15011,.F.);
#20277=ORIENTED_EDGE('',*,*,#15010,.F.);
#20278=ORIENTED_EDGE('',*,*,#15012,.T.);
#20279=ORIENTED_EDGE('',*,*,#15013,.F.);
#20280=ORIENTED_EDGE('',*,*,#15012,.F.);
#20281=ORIENTED_EDGE('',*,*,#15014,.T.);
#20282=ORIENTED_EDGE('',*,*,#15015,.T.);
#20283=ORIENTED_EDGE('',*,*,#14989,.T.);
#20284=ORIENTED_EDGE('',*,*,#15015,.F.);
#20285=ORIENTED_EDGE('',*,*,#15014,.F.);
#20286=ORIENTED_EDGE('',*,*,#15016,.T.);
#20287=ORIENTED_EDGE('',*,*,#15017,.F.);
#20288=ORIENTED_EDGE('',*,*,#15016,.F.);
#20289=ORIENTED_EDGE('',*,*,#15018,.T.);
#20290=ORIENTED_EDGE('',*,*,#15019,.T.);
#20291=ORIENTED_EDGE('',*,*,#14975,.T.);
#20292=ORIENTED_EDGE('',*,*,#15019,.F.);
#20293=ORIENTED_EDGE('',*,*,#15018,.F.);
#20294=ORIENTED_EDGE('',*,*,#15020,.T.);
#20295=ORIENTED_EDGE('',*,*,#15021,.F.);
#20296=ORIENTED_EDGE('',*,*,#15020,.F.);
#20297=ORIENTED_EDGE('',*,*,#15022,.T.);
#20298=ORIENTED_EDGE('',*,*,#15023,.T.);
#20299=ORIENTED_EDGE('',*,*,#14988,.T.);
#20300=ORIENTED_EDGE('',*,*,#15023,.F.);
#20301=ORIENTED_EDGE('',*,*,#15022,.F.);
#20302=ORIENTED_EDGE('',*,*,#15024,.T.);
#20303=ORIENTED_EDGE('',*,*,#15025,.F.);
#20304=ORIENTED_EDGE('',*,*,#15024,.F.);
#20305=ORIENTED_EDGE('',*,*,#15026,.T.);
#20306=ORIENTED_EDGE('',*,*,#15027,.T.);
#20307=ORIENTED_EDGE('',*,*,#14976,.T.);
#20308=ORIENTED_EDGE('',*,*,#15027,.F.);
#20309=ORIENTED_EDGE('',*,*,#15026,.F.);
#20310=ORIENTED_EDGE('',*,*,#15028,.T.);
#20311=ORIENTED_EDGE('',*,*,#15029,.F.);
#20312=ORIENTED_EDGE('',*,*,#15028,.F.);
#20313=ORIENTED_EDGE('',*,*,#15030,.T.);
#20314=ORIENTED_EDGE('',*,*,#15031,.T.);
#20315=ORIENTED_EDGE('',*,*,#14987,.T.);
#20316=ORIENTED_EDGE('',*,*,#15031,.F.);
#20317=ORIENTED_EDGE('',*,*,#15030,.F.);
#20318=ORIENTED_EDGE('',*,*,#15032,.T.);
#20319=ORIENTED_EDGE('',*,*,#15033,.F.);
#20320=ORIENTED_EDGE('',*,*,#15032,.F.);
#20321=ORIENTED_EDGE('',*,*,#15034,.T.);
#20322=ORIENTED_EDGE('',*,*,#15035,.T.);
#20323=ORIENTED_EDGE('',*,*,#14977,.T.);
#20324=ORIENTED_EDGE('',*,*,#15035,.F.);
#20325=ORIENTED_EDGE('',*,*,#15034,.F.);
#20326=ORIENTED_EDGE('',*,*,#15036,.T.);
#20327=ORIENTED_EDGE('',*,*,#15037,.F.);
#20328=ORIENTED_EDGE('',*,*,#15036,.F.);
#20329=ORIENTED_EDGE('',*,*,#15038,.T.);
#20330=ORIENTED_EDGE('',*,*,#15039,.T.);
#20331=ORIENTED_EDGE('',*,*,#14986,.T.);
#20332=ORIENTED_EDGE('',*,*,#15039,.F.);
#20333=ORIENTED_EDGE('',*,*,#15038,.F.);
#20334=ORIENTED_EDGE('',*,*,#15040,.T.);
#20335=ORIENTED_EDGE('',*,*,#15041,.F.);
#20336=ORIENTED_EDGE('',*,*,#15040,.F.);
#20337=ORIENTED_EDGE('',*,*,#15042,.T.);
#20338=ORIENTED_EDGE('',*,*,#15043,.T.);
#20339=ORIENTED_EDGE('',*,*,#14978,.T.);
#20340=ORIENTED_EDGE('',*,*,#15043,.F.);
#20341=ORIENTED_EDGE('',*,*,#15042,.F.);
#20342=ORIENTED_EDGE('',*,*,#15044,.T.);
#20343=ORIENTED_EDGE('',*,*,#15045,.F.);
#20344=ORIENTED_EDGE('',*,*,#15044,.F.);
#20345=ORIENTED_EDGE('',*,*,#15046,.T.);
#20346=ORIENTED_EDGE('',*,*,#15047,.T.);
#20347=ORIENTED_EDGE('',*,*,#14985,.T.);
#20348=ORIENTED_EDGE('',*,*,#15047,.F.);
#20349=ORIENTED_EDGE('',*,*,#15046,.F.);
#20350=ORIENTED_EDGE('',*,*,#15048,.T.);
#20351=ORIENTED_EDGE('',*,*,#15049,.F.);
#20352=ORIENTED_EDGE('',*,*,#15048,.F.);
#20353=ORIENTED_EDGE('',*,*,#15050,.T.);
#20354=ORIENTED_EDGE('',*,*,#15051,.T.);
#20355=ORIENTED_EDGE('',*,*,#14979,.T.);
#20356=ORIENTED_EDGE('',*,*,#15051,.F.);
#20357=ORIENTED_EDGE('',*,*,#15050,.F.);
#20358=ORIENTED_EDGE('',*,*,#15052,.T.);
#20359=ORIENTED_EDGE('',*,*,#15053,.F.);
#20360=ORIENTED_EDGE('',*,*,#15052,.F.);
#20361=ORIENTED_EDGE('',*,*,#15054,.T.);
#20362=ORIENTED_EDGE('',*,*,#15055,.T.);
#20363=ORIENTED_EDGE('',*,*,#14984,.T.);
#20364=ORIENTED_EDGE('',*,*,#15055,.F.);
#20365=ORIENTED_EDGE('',*,*,#15054,.F.);
#20366=ORIENTED_EDGE('',*,*,#15056,.T.);
#20367=ORIENTED_EDGE('',*,*,#15057,.F.);
#20368=ORIENTED_EDGE('',*,*,#15056,.F.);
#20369=ORIENTED_EDGE('',*,*,#15058,.T.);
#20370=ORIENTED_EDGE('',*,*,#15059,.T.);
#20371=ORIENTED_EDGE('',*,*,#14980,.T.);
#20372=ORIENTED_EDGE('',*,*,#15059,.F.);
#20373=ORIENTED_EDGE('',*,*,#15058,.F.);
#20374=ORIENTED_EDGE('',*,*,#15060,.T.);
#20375=ORIENTED_EDGE('',*,*,#15061,.F.);
#20376=ORIENTED_EDGE('',*,*,#15060,.F.);
#20377=ORIENTED_EDGE('',*,*,#15062,.T.);
#20378=ORIENTED_EDGE('',*,*,#15063,.T.);
#20379=ORIENTED_EDGE('',*,*,#14983,.T.);
#20380=ORIENTED_EDGE('',*,*,#15063,.F.);
#20381=ORIENTED_EDGE('',*,*,#15062,.F.);
#20382=ORIENTED_EDGE('',*,*,#15064,.T.);
#20383=ORIENTED_EDGE('',*,*,#15065,.F.);
#20384=ORIENTED_EDGE('',*,*,#15064,.F.);
#20385=ORIENTED_EDGE('',*,*,#15066,.T.);
#20386=ORIENTED_EDGE('',*,*,#15067,.T.);
#20387=ORIENTED_EDGE('',*,*,#14981,.T.);
#20388=ORIENTED_EDGE('',*,*,#15067,.F.);
#20389=ORIENTED_EDGE('',*,*,#15066,.F.);
#20390=ORIENTED_EDGE('',*,*,#15068,.T.);
#20391=ORIENTED_EDGE('',*,*,#15069,.F.);
#20392=ORIENTED_EDGE('',*,*,#15068,.F.);
#20393=ORIENTED_EDGE('',*,*,#15070,.T.);
#20394=ORIENTED_EDGE('',*,*,#15071,.T.);
#20395=ORIENTED_EDGE('',*,*,#14982,.T.);
#20396=ORIENTED_EDGE('',*,*,#15071,.F.);
#20397=ORIENTED_EDGE('',*,*,#15070,.F.);
#20398=ORIENTED_EDGE('',*,*,#15072,.T.);
#20399=ORIENTED_EDGE('',*,*,#15073,.F.);
#20400=ORIENTED_EDGE('',*,*,#15072,.F.);
#20401=ORIENTED_EDGE('',*,*,#15074,.T.);
#20402=ORIENTED_EDGE('',*,*,#14968,.T.);
#20403=ORIENTED_EDGE('',*,*,#15075,.T.);
#20404=ORIENTED_EDGE('',*,*,#15076,.T.);
#20405=ORIENTED_EDGE('',*,*,#15077,.T.);
#20406=ORIENTED_EDGE('',*,*,#14969,.T.);
#20407=ORIENTED_EDGE('',*,*,#15074,.F.);
#20408=ORIENTED_EDGE('',*,*,#15078,.T.);
#20409=ORIENTED_EDGE('',*,*,#15079,.T.);
#20410=ORIENTED_EDGE('',*,*,#14970,.T.);
#20411=ORIENTED_EDGE('',*,*,#15077,.F.);
#20412=ORIENTED_EDGE('',*,*,#15080,.T.);
#20413=ORIENTED_EDGE('',*,*,#15075,.F.);
#20414=ORIENTED_EDGE('',*,*,#14971,.T.);
#20415=ORIENTED_EDGE('',*,*,#15079,.F.);
#20416=ORIENTED_EDGE('',*,*,#15081,.T.);
#20417=ORIENTED_EDGE('',*,*,#15078,.F.);
#20418=ORIENTED_EDGE('',*,*,#15082,.F.);
#20419=ORIENTED_EDGE('',*,*,#15083,.F.);
#20420=ORIENTED_EDGE('',*,*,#15084,.T.);
#20421=ORIENTED_EDGE('',*,*,#15076,.F.);
#20422=ORIENTED_EDGE('',*,*,#15085,.F.);
#20423=ORIENTED_EDGE('',*,*,#15086,.F.);
#20424=ORIENTED_EDGE('',*,*,#15082,.T.);
#20425=ORIENTED_EDGE('',*,*,#15087,.T.);
#20426=ORIENTED_EDGE('',*,*,#15088,.T.);
#20427=ORIENTED_EDGE('',*,*,#15089,.T.);
#20428=ORIENTED_EDGE('',*,*,#15086,.T.);
#20429=ORIENTED_EDGE('',*,*,#15087,.F.);
#20430=ORIENTED_EDGE('',*,*,#15090,.T.);
#20431=ORIENTED_EDGE('',*,*,#15091,.T.);
#20432=ORIENTED_EDGE('',*,*,#15092,.T.);
#20433=ORIENTED_EDGE('',*,*,#15093,.T.);
#20434=ORIENTED_EDGE('',*,*,#15094,.T.);
#20435=ORIENTED_EDGE('',*,*,#15091,.F.);
#20436=ORIENTED_EDGE('',*,*,#15095,.T.);
#20437=ORIENTED_EDGE('',*,*,#15093,.F.);
#20438=ORIENTED_EDGE('',*,*,#15083,.T.);
#20439=ORIENTED_EDGE('',*,*,#15089,.F.);
#20440=ORIENTED_EDGE('',*,*,#15096,.T.);
#20441=ORIENTED_EDGE('',*,*,#15081,.F.);
#20442=ORIENTED_EDGE('',*,*,#15097,.F.);
#20443=ORIENTED_EDGE('',*,*,#15090,.F.);
#20444=ORIENTED_EDGE('',*,*,#15085,.T.);
#20445=ORIENTED_EDGE('',*,*,#15088,.F.);
#20446=ORIENTED_EDGE('',*,*,#15092,.F.);
#20447=ORIENTED_EDGE('',*,*,#15094,.F.);
#20448=ORIENTED_EDGE('',*,*,#15096,.F.);
#20449=ORIENTED_EDGE('',*,*,#14993,.T.);
#20450=ORIENTED_EDGE('',*,*,#14997,.T.);
#20451=ORIENTED_EDGE('',*,*,#15001,.T.);
#20452=ORIENTED_EDGE('',*,*,#15005,.T.);
#20453=ORIENTED_EDGE('',*,*,#15009,.T.);
#20454=ORIENTED_EDGE('',*,*,#15013,.T.);
#20455=ORIENTED_EDGE('',*,*,#15017,.T.);
#20456=ORIENTED_EDGE('',*,*,#15021,.T.);
#20457=ORIENTED_EDGE('',*,*,#15025,.T.);
#20458=ORIENTED_EDGE('',*,*,#15029,.T.);
#20459=ORIENTED_EDGE('',*,*,#15033,.T.);
#20460=ORIENTED_EDGE('',*,*,#15037,.T.);
#20461=ORIENTED_EDGE('',*,*,#15041,.T.);
#20462=ORIENTED_EDGE('',*,*,#15045,.T.);
#20463=ORIENTED_EDGE('',*,*,#15049,.T.);
#20464=ORIENTED_EDGE('',*,*,#15053,.T.);
#20465=ORIENTED_EDGE('',*,*,#15057,.T.);
#20466=ORIENTED_EDGE('',*,*,#15061,.T.);
#20467=ORIENTED_EDGE('',*,*,#15065,.T.);
#20468=ORIENTED_EDGE('',*,*,#15069,.T.);
#20469=ORIENTED_EDGE('',*,*,#15073,.T.);
#20470=ORIENTED_EDGE('',*,*,#15080,.F.);
#20471=ORIENTED_EDGE('',*,*,#15084,.F.);
#20472=ORIENTED_EDGE('',*,*,#15095,.F.);
#20473=ORIENTED_EDGE('',*,*,#15097,.T.);
#25489=CONICAL_SURFACE('',#27873,1.87799999999999,0.785398163397448);
#25490=CONICAL_SURFACE('',#27901,1.87799999999999,0.785398163397448);
#25491=CONICAL_SURFACE('',#27905,1.878,0.785398163397448);
#25492=CONICAL_SURFACE('',#27909,1.878,0.785398163397448);
#25493=CONICAL_SURFACE('',#27913,1.878,0.785398163397459);
#25494=CONICAL_SURFACE('',#27917,1.87799999999999,0.785398163397448);
#25495=CONICAL_SURFACE('',#27921,1.878,0.785398163397459);
#25496=CONICAL_SURFACE('',#27925,1.878,0.785398163397459);
#25497=CONICAL_SURFACE('',#27929,1.878,0.785398163397448);
#25498=CONICAL_SURFACE('',#27933,1.878,0.785398163397448);
#25499=CONICAL_SURFACE('',#27937,1.87799999999999,0.785398163397448);
#25500=CONICAL_SURFACE('',#27941,1.878,0.785398163397448);
#25501=CONICAL_SURFACE('',#27945,1.878,0.785398163397448);
#25502=CONICAL_SURFACE('',#27949,1.878,0.785398163397459);
#25503=CONICAL_SURFACE('',#27953,1.878,0.785398163397459);
#25504=CONICAL_SURFACE('',#27957,1.878,0.785398163397459);
#25505=CONICAL_SURFACE('',#27961,1.878,0.785398163397459);
#25506=CONICAL_SURFACE('',#27965,1.878,0.785398163397459);
#25507=CONICAL_SURFACE('',#27969,1.878,0.785398163397448);
#25508=CONICAL_SURFACE('',#27973,1.878,0.785398163397448);
#25509=CONICAL_SURFACE('',#27977,1.87799999999999,0.785398163397448);
#25510=CONICAL_SURFACE('',#27982,4.6375,0.785398163397448);
#25511=CONICAL_SURFACE('',#27985,4.6375,0.785398163397448);
#25512=CONICAL_SURFACE('',#27991,4.6375,0.785398163397448);
#25513=CONICAL_SURFACE('',#27995,4.6375,0.785398163397448);
#26034=ADVANCED_FACE('',(#2841),#25489,.F.);
#26035=ADVANCED_FACE('',(#2842,#1019,#1020,#1021,#1022,#1023,#1024,#1025,
#1026,#1027,#1028,#1029,#1030,#1031,#1032,#1033,#1034,#1035,#1036,#1037,
#1038,#1039),#1415,.T.);
#26036=ADVANCED_FACE('',(#2843),#2259,.F.);
#26037=ADVANCED_FACE('',(#2844),#25490,.F.);
#26038=ADVANCED_FACE('',(#2845),#2260,.F.);
#26039=ADVANCED_FACE('',(#2846),#25491,.F.);
#26040=ADVANCED_FACE('',(#2847),#2261,.F.);
#26041=ADVANCED_FACE('',(#2848),#25492,.F.);
#26042=ADVANCED_FACE('',(#2849),#2262,.F.);
#26043=ADVANCED_FACE('',(#2850),#25493,.F.);
#26044=ADVANCED_FACE('',(#2851),#2263,.F.);
#26045=ADVANCED_FACE('',(#2852),#25494,.F.);
#26046=ADVANCED_FACE('',(#2853),#2264,.F.);
#26047=ADVANCED_FACE('',(#2854),#25495,.F.);
#26048=ADVANCED_FACE('',(#2855),#2265,.F.);
#26049=ADVANCED_FACE('',(#2856),#25496,.F.);
#26050=ADVANCED_FACE('',(#2857),#2266,.F.);
#26051=ADVANCED_FACE('',(#2858),#25497,.F.);
#26052=ADVANCED_FACE('',(#2859),#2267,.F.);
#26053=ADVANCED_FACE('',(#2860),#25498,.F.);
#26054=ADVANCED_FACE('',(#2861),#2268,.F.);
#26055=ADVANCED_FACE('',(#2862),#25499,.F.);
#26056=ADVANCED_FACE('',(#2863),#2269,.F.);
#26057=ADVANCED_FACE('',(#2864),#25500,.F.);
#26058=ADVANCED_FACE('',(#2865),#2270,.F.);
#26059=ADVANCED_FACE('',(#2866),#25501,.F.);
#26060=ADVANCED_FACE('',(#2867),#2271,.F.);
#26061=ADVANCED_FACE('',(#2868),#25502,.F.);
#26062=ADVANCED_FACE('',(#2869),#2272,.F.);
#26063=ADVANCED_FACE('',(#2870),#25503,.F.);
#26064=ADVANCED_FACE('',(#2871),#2273,.F.);
#26065=ADVANCED_FACE('',(#2872),#25504,.F.);
#26066=ADVANCED_FACE('',(#2873),#2274,.F.);
#26067=ADVANCED_FACE('',(#2874),#25505,.F.);
#26068=ADVANCED_FACE('',(#2875),#2275,.F.);
#26069=ADVANCED_FACE('',(#2876),#25506,.F.);
#26070=ADVANCED_FACE('',(#2877),#2276,.F.);
#26071=ADVANCED_FACE('',(#2878),#25507,.F.);
#26072=ADVANCED_FACE('',(#2879),#2277,.F.);
#26073=ADVANCED_FACE('',(#2880),#25508,.F.);
#26074=ADVANCED_FACE('',(#2881),#2278,.F.);
#26075=ADVANCED_FACE('',(#2882),#25509,.F.);
#26076=ADVANCED_FACE('',(#2883),#2279,.F.);
#26077=ADVANCED_FACE('',(#2884),#1416,.T.);
#26078=ADVANCED_FACE('',(#2885),#25510,.T.);
#26079=ADVANCED_FACE('',(#2886),#1417,.T.);
#26080=ADVANCED_FACE('',(#2887),#25511,.T.);
#26081=ADVANCED_FACE('',(#2888),#2280,.T.);
#26082=ADVANCED_FACE('',(#2889),#1418,.T.);
#26083=ADVANCED_FACE('',(#2890),#1419,.T.);
#26084=ADVANCED_FACE('',(#2891),#25512,.T.);
#26085=ADVANCED_FACE('',(#2892),#1420,.T.);
#26086=ADVANCED_FACE('',(#2893),#25513,.T.);
#26087=ADVANCED_FACE('',(#2894),#2281,.T.);
#26088=ADVANCED_FACE('',(#2895,#1040,#1041,#1042,#1043,#1044,#1045,#1046,
#1047,#1048,#1049,#1050,#1051,#1052,#1053,#1054,#1055,#1056,#1057,#1058,
#1059,#1060),#1421,.F.);
#26089=ADVANCED_FACE('',(#2896),#1422,.T.);
#26934=CLOSED_SHELL('',(#26034,#26035,#26036,#26037,#26038,#26039,#26040,
#26041,#26042,#26043,#26044,#26045,#26046,#26047,#26048,#26049,#26050,#26051,
#26052,#26053,#26054,#26055,#26056,#26057,#26058,#26059,#26060,#26061,#26062,
#26063,#26064,#26065,#26066,#26067,#26068,#26069,#26070,#26071,#26072,#26073,
#26074,#26075,#26076,#26077,#26078,#26079,#26080,#26081,#26082,#26083,#26084,
#26085,#26086,#26087,#26088,#26089));
#27872=AXIS2_PLACEMENT_3D('',#50671,#31579,#31580);
#27873=AXIS2_PLACEMENT_3D('',#50672,#31581,#31582);
#27874=AXIS2_PLACEMENT_3D('',#50674,#31583,#31584);
#27875=AXIS2_PLACEMENT_3D('',#50677,#31586,#31587);
#27876=AXIS2_PLACEMENT_3D('',#50678,#31588,#31589);
#27877=AXIS2_PLACEMENT_3D('',#50683,#31591,#31592);
#27878=AXIS2_PLACEMENT_3D('',#50686,#31594,#31595);
#27879=AXIS2_PLACEMENT_3D('',#50688,#31596,#31597);
#27880=AXIS2_PLACEMENT_3D('',#50690,#31598,#31599);
#27881=AXIS2_PLACEMENT_3D('',#50692,#31600,#31601);
#27882=AXIS2_PLACEMENT_3D('',#50694,#31602,#31603);
#27883=AXIS2_PLACEMENT_3D('',#50696,#31604,#31605);
#27884=AXIS2_PLACEMENT_3D('',#50698,#31606,#31607);
#27885=AXIS2_PLACEMENT_3D('',#50700,#31608,#31609);
#27886=AXIS2_PLACEMENT_3D('',#50702,#31610,#31611);
#27887=AXIS2_PLACEMENT_3D('',#50704,#31612,#31613);
#27888=AXIS2_PLACEMENT_3D('',#50706,#31614,#31615);
#27889=AXIS2_PLACEMENT_3D('',#50708,#31616,#31617);
#27890=AXIS2_PLACEMENT_3D('',#50710,#31618,#31619);
#27891=AXIS2_PLACEMENT_3D('',#50712,#31620,#31621);
#27892=AXIS2_PLACEMENT_3D('',#50714,#31622,#31623);
#27893=AXIS2_PLACEMENT_3D('',#50716,#31624,#31625);
#27894=AXIS2_PLACEMENT_3D('',#50718,#31626,#31627);
#27895=AXIS2_PLACEMENT_3D('',#50720,#31628,#31629);
#27896=AXIS2_PLACEMENT_3D('',#50722,#31630,#31631);
#27897=AXIS2_PLACEMENT_3D('',#50724,#31632,#31633);
#27898=AXIS2_PLACEMENT_3D('',#50726,#31634,#31635);
#27899=AXIS2_PLACEMENT_3D('',#50727,#31636,#31637);
#27900=AXIS2_PLACEMENT_3D('',#50730,#31639,#31640);
#27901=AXIS2_PLACEMENT_3D('',#50731,#31641,#31642);
#27902=AXIS2_PLACEMENT_3D('',#50733,#31643,#31644);
#27903=AXIS2_PLACEMENT_3D('',#50735,#31646,#31647);
#27904=AXIS2_PLACEMENT_3D('',#50738,#31649,#31650);
#27905=AXIS2_PLACEMENT_3D('',#50739,#31651,#31652);
#27906=AXIS2_PLACEMENT_3D('',#50741,#31653,#31654);
#27907=AXIS2_PLACEMENT_3D('',#50743,#31656,#31657);
#27908=AXIS2_PLACEMENT_3D('',#50746,#31659,#31660);
#27909=AXIS2_PLACEMENT_3D('',#50747,#31661,#31662);
#27910=AXIS2_PLACEMENT_3D('',#50749,#31663,#31664);
#27911=AXIS2_PLACEMENT_3D('',#50751,#31666,#31667);
#27912=AXIS2_PLACEMENT_3D('',#50754,#31669,#31670);
#27913=AXIS2_PLACEMENT_3D('',#50755,#31671,#31672);
#27914=AXIS2_PLACEMENT_3D('',#50757,#31673,#31674);
#27915=AXIS2_PLACEMENT_3D('',#50759,#31676,#31677);
#27916=AXIS2_PLACEMENT_3D('',#50762,#31679,#31680);
#27917=AXIS2_PLACEMENT_3D('',#50763,#31681,#31682);
#27918=AXIS2_PLACEMENT_3D('',#50765,#31683,#31684);
#27919=AXIS2_PLACEMENT_3D('',#50767,#31686,#31687);
#27920=AXIS2_PLACEMENT_3D('',#50770,#31689,#31690);
#27921=AXIS2_PLACEMENT_3D('',#50771,#31691,#31692);
#27922=AXIS2_PLACEMENT_3D('',#50773,#31693,#31694);
#27923=AXIS2_PLACEMENT_3D('',#50775,#31696,#31697);
#27924=AXIS2_PLACEMENT_3D('',#50778,#31699,#31700);
#27925=AXIS2_PLACEMENT_3D('',#50779,#31701,#31702);
#27926=AXIS2_PLACEMENT_3D('',#50781,#31703,#31704);
#27927=AXIS2_PLACEMENT_3D('',#50783,#31706,#31707);
#27928=AXIS2_PLACEMENT_3D('',#50786,#31709,#31710);
#27929=AXIS2_PLACEMENT_3D('',#50787,#31711,#31712);
#27930=AXIS2_PLACEMENT_3D('',#50789,#31713,#31714);
#27931=AXIS2_PLACEMENT_3D('',#50791,#31716,#31717);
#27932=AXIS2_PLACEMENT_3D('',#50794,#31719,#31720);
#27933=AXIS2_PLACEMENT_3D('',#50795,#31721,#31722);
#27934=AXIS2_PLACEMENT_3D('',#50797,#31723,#31724);
#27935=AXIS2_PLACEMENT_3D('',#50799,#31726,#31727);
#27936=AXIS2_PLACEMENT_3D('',#50802,#31729,#31730);
#27937=AXIS2_PLACEMENT_3D('',#50803,#31731,#31732);
#27938=AXIS2_PLACEMENT_3D('',#50805,#31733,#31734);
#27939=AXIS2_PLACEMENT_3D('',#50807,#31736,#31737);
#27940=AXIS2_PLACEMENT_3D('',#50810,#31739,#31740);
#27941=AXIS2_PLACEMENT_3D('',#50811,#31741,#31742);
#27942=AXIS2_PLACEMENT_3D('',#50813,#31743,#31744);
#27943=AXIS2_PLACEMENT_3D('',#50815,#31746,#31747);
#27944=AXIS2_PLACEMENT_3D('',#50818,#31749,#31750);
#27945=AXIS2_PLACEMENT_3D('',#50819,#31751,#31752);
#27946=AXIS2_PLACEMENT_3D('',#50821,#31753,#31754);
#27947=AXIS2_PLACEMENT_3D('',#50823,#31756,#31757);
#27948=AXIS2_PLACEMENT_3D('',#50826,#31759,#31760);
#27949=AXIS2_PLACEMENT_3D('',#50827,#31761,#31762);
#27950=AXIS2_PLACEMENT_3D('',#50829,#31763,#31764);
#27951=AXIS2_PLACEMENT_3D('',#50831,#31766,#31767);
#27952=AXIS2_PLACEMENT_3D('',#50834,#31769,#31770);
#27953=AXIS2_PLACEMENT_3D('',#50835,#31771,#31772);
#27954=AXIS2_PLACEMENT_3D('',#50837,#31773,#31774);
#27955=AXIS2_PLACEMENT_3D('',#50839,#31776,#31777);
#27956=AXIS2_PLACEMENT_3D('',#50842,#31779,#31780);
#27957=AXIS2_PLACEMENT_3D('',#50843,#31781,#31782);
#27958=AXIS2_PLACEMENT_3D('',#50845,#31783,#31784);
#27959=AXIS2_PLACEMENT_3D('',#50847,#31786,#31787);
#27960=AXIS2_PLACEMENT_3D('',#50850,#31789,#31790);
#27961=AXIS2_PLACEMENT_3D('',#50851,#31791,#31792);
#27962=AXIS2_PLACEMENT_3D('',#50853,#31793,#31794);
#27963=AXIS2_PLACEMENT_3D('',#50855,#31796,#31797);
#27964=AXIS2_PLACEMENT_3D('',#50858,#31799,#31800);
#27965=AXIS2_PLACEMENT_3D('',#50859,#31801,#31802);
#27966=AXIS2_PLACEMENT_3D('',#50861,#31803,#31804);
#27967=AXIS2_PLACEMENT_3D('',#50863,#31806,#31807);
#27968=AXIS2_PLACEMENT_3D('',#50866,#31809,#31810);
#27969=AXIS2_PLACEMENT_3D('',#50867,#31811,#31812);
#27970=AXIS2_PLACEMENT_3D('',#50869,#31813,#31814);
#27971=AXIS2_PLACEMENT_3D('',#50871,#31816,#31817);
#27972=AXIS2_PLACEMENT_3D('',#50874,#31819,#31820);
#27973=AXIS2_PLACEMENT_3D('',#50875,#31821,#31822);
#27974=AXIS2_PLACEMENT_3D('',#50877,#31823,#31824);
#27975=AXIS2_PLACEMENT_3D('',#50879,#31826,#31827);
#27976=AXIS2_PLACEMENT_3D('',#50882,#31829,#31830);
#27977=AXIS2_PLACEMENT_3D('',#50883,#31831,#31832);
#27978=AXIS2_PLACEMENT_3D('',#50885,#31833,#31834);
#27979=AXIS2_PLACEMENT_3D('',#50887,#31836,#31837);
#27980=AXIS2_PLACEMENT_3D('',#50890,#31839,#31840);
#27981=AXIS2_PLACEMENT_3D('',#50891,#31841,#31842);
#27982=AXIS2_PLACEMENT_3D('',#50897,#31846,#31847);
#27983=AXIS2_PLACEMENT_3D('',#50900,#31849,#31850);
#27984=AXIS2_PLACEMENT_3D('',#50901,#31851,#31852);
#27985=AXIS2_PLACEMENT_3D('',#50905,#31855,#31856);
#27986=AXIS2_PLACEMENT_3D('',#50906,#31857,#31858);
#27987=AXIS2_PLACEMENT_3D('',#50907,#31859,#31860);
#27988=AXIS2_PLACEMENT_3D('',#50911,#31862,#31863);
#27989=AXIS2_PLACEMENT_3D('',#50913,#31865,#31866);
#27990=AXIS2_PLACEMENT_3D('',#50917,#31869,#31870);
#27991=AXIS2_PLACEMENT_3D('',#50923,#31874,#31875);
#27992=AXIS2_PLACEMENT_3D('',#50925,#31876,#31877);
#27993=AXIS2_PLACEMENT_3D('',#50928,#31879,#31880);
#27994=AXIS2_PLACEMENT_3D('',#50929,#31881,#31882);
#27995=AXIS2_PLACEMENT_3D('',#50934,#31886,#31887);
#27996=AXIS2_PLACEMENT_3D('',#50935,#31888,#31889);
#27997=AXIS2_PLACEMENT_3D('',#50936,#31890,#31891);
#27998=AXIS2_PLACEMENT_3D('',#50938,#31893,#31894);
#27999=AXIS2_PLACEMENT_3D('',#50939,#31895,#31896);
#31579=DIRECTION('axis',(0.,0.,1.));
#31580=DIRECTION('refdir',(1.,0.,0.));
#31581=DIRECTION('center_axis',(0.,1.,0.));
#31582=DIRECTION('ref_axis',(1.,0.,0.));
#31583=DIRECTION('center_axis',(0.,-1.,0.));
#31584=DIRECTION('ref_axis',(1.,0.,0.));
#31585=DIRECTION('',(-0.707106781186547,0.707106781186548,8.65956056235493E-17));
#31586=DIRECTION('center_axis',(0.,1.,0.));
#31587=DIRECTION('ref_axis',(1.,0.,0.));
#31588=DIRECTION('center_axis',(0.,1.,0.));
#31589=DIRECTION('ref_axis',(1.,0.,0.));
#31590=DIRECTION('',(-1.,0.,0.));
#31591=DIRECTION('center_axis',(0.,-1.,0.));
#31592=DIRECTION('ref_axis',(0.,0.,1.));
#31593=DIRECTION('',(1.,0.,0.));
#31594=DIRECTION('center_axis',(0.,-1.,0.));
#31595=DIRECTION('ref_axis',(0.,0.,-1.));
#31596=DIRECTION('center_axis',(0.,1.,0.));
#31597=DIRECTION('ref_axis',(1.,0.,0.));
#31598=DIRECTION('center_axis',(0.,1.,0.));
#31599=DIRECTION('ref_axis',(1.,0.,0.));
#31600=DIRECTION('center_axis',(0.,1.,0.));
#31601=DIRECTION('ref_axis',(1.,0.,0.));
#31602=DIRECTION('center_axis',(0.,1.,0.));
#31603=DIRECTION('ref_axis',(1.,0.,0.));
#31604=DIRECTION('center_axis',(0.,1.,0.));
#31605=DIRECTION('ref_axis',(1.,0.,0.));
#31606=DIRECTION('center_axis',(0.,1.,0.));
#31607=DIRECTION('ref_axis',(1.,0.,0.));
#31608=DIRECTION('center_axis',(0.,1.,0.));
#31609=DIRECTION('ref_axis',(1.,0.,0.));
#31610=DIRECTION('center_axis',(0.,1.,0.));
#31611=DIRECTION('ref_axis',(1.,0.,0.));
#31612=DIRECTION('center_axis',(0.,1.,0.));
#31613=DIRECTION('ref_axis',(1.,0.,0.));
#31614=DIRECTION('center_axis',(0.,1.,0.));
#31615=DIRECTION('ref_axis',(1.,0.,0.));
#31616=DIRECTION('center_axis',(0.,1.,0.));
#31617=DIRECTION('ref_axis',(1.,0.,0.));
#31618=DIRECTION('center_axis',(0.,1.,0.));
#31619=DIRECTION('ref_axis',(1.,0.,0.));
#31620=DIRECTION('center_axis',(0.,1.,0.));
#31621=DIRECTION('ref_axis',(1.,0.,0.));
#31622=DIRECTION('center_axis',(0.,1.,0.));
#31623=DIRECTION('ref_axis',(1.,0.,0.));
#31624=DIRECTION('center_axis',(0.,1.,0.));
#31625=DIRECTION('ref_axis',(1.,0.,0.));
#31626=DIRECTION('center_axis',(0.,1.,0.));
#31627=DIRECTION('ref_axis',(1.,0.,0.));
#31628=DIRECTION('center_axis',(0.,1.,0.));
#31629=DIRECTION('ref_axis',(1.,0.,0.));
#31630=DIRECTION('center_axis',(0.,1.,0.));
#31631=DIRECTION('ref_axis',(1.,0.,0.));
#31632=DIRECTION('center_axis',(0.,1.,0.));
#31633=DIRECTION('ref_axis',(1.,0.,0.));
#31634=DIRECTION('center_axis',(0.,1.,0.));
#31635=DIRECTION('ref_axis',(1.,0.,0.));
#31636=DIRECTION('center_axis',(0.,-1.,0.));
#31637=DIRECTION('ref_axis',(1.,0.,0.));
#31638=DIRECTION('',(0.,-1.,0.));
#31639=DIRECTION('center_axis',(0.,1.,0.));
#31640=DIRECTION('ref_axis',(1.,0.,0.));
#31641=DIRECTION('center_axis',(0.,1.,0.));
#31642=DIRECTION('ref_axis',(1.,0.,0.));
#31643=DIRECTION('center_axis',(0.,-1.,0.));
#31644=DIRECTION('ref_axis',(1.,0.,0.));
#31645=DIRECTION('',(-0.707106781186547,0.707106781186548,8.65956056235493E-17));
#31646=DIRECTION('center_axis',(0.,-1.,0.));
#31647=DIRECTION('ref_axis',(1.,0.,0.));
#31648=DIRECTION('',(0.,-1.,0.));
#31649=DIRECTION('center_axis',(0.,1.,0.));
#31650=DIRECTION('ref_axis',(1.,0.,0.));
#31651=DIRECTION('center_axis',(0.,1.,0.));
#31652=DIRECTION('ref_axis',(1.,0.,0.));
#31653=DIRECTION('center_axis',(0.,-1.,0.));
#31654=DIRECTION('ref_axis',(1.,0.,0.));
#31655=DIRECTION('',(-0.707106781186547,0.707106781186548,8.65956056235493E-17));
#31656=DIRECTION('center_axis',(0.,-1.,0.));
#31657=DIRECTION('ref_axis',(1.,0.,0.));
#31658=DIRECTION('',(0.,-1.,0.));
#31659=DIRECTION('center_axis',(0.,1.,0.));
#31660=DIRECTION('ref_axis',(1.,0.,0.));
#31661=DIRECTION('center_axis',(0.,1.,0.));
#31662=DIRECTION('ref_axis',(1.,0.,0.));
#31663=DIRECTION('center_axis',(0.,-1.,0.));
#31664=DIRECTION('ref_axis',(1.,0.,0.));
#31665=DIRECTION('',(-0.707106781186547,0.707106781186548,8.65956056235493E-17));
#31666=DIRECTION('center_axis',(0.,-1.,0.));
#31667=DIRECTION('ref_axis',(1.,0.,0.));
#31668=DIRECTION('',(0.,-1.,0.));
#31669=DIRECTION('center_axis',(0.,1.,0.));
#31670=DIRECTION('ref_axis',(1.,0.,0.));
#31671=DIRECTION('center_axis',(0.,1.,0.));
#31672=DIRECTION('ref_axis',(1.,0.,0.));
#31673=DIRECTION('center_axis',(0.,-1.,0.));
#31674=DIRECTION('ref_axis',(1.,0.,0.));
#31675=DIRECTION('',(-0.707106781186555,0.70710678118654,8.65956056235503E-17));
#31676=DIRECTION('center_axis',(0.,-1.,0.));
#31677=DIRECTION('ref_axis',(1.,0.,0.));
#31678=DIRECTION('',(0.,-1.,0.));
#31679=DIRECTION('center_axis',(0.,1.,0.));
#31680=DIRECTION('ref_axis',(1.,0.,0.));
#31681=DIRECTION('center_axis',(0.,1.,0.));
#31682=DIRECTION('ref_axis',(1.,0.,0.));
#31683=DIRECTION('center_axis',(0.,-1.,0.));
#31684=DIRECTION('ref_axis',(1.,0.,0.));
#31685=DIRECTION('',(-0.707106781186547,0.707106781186548,8.65956056235493E-17));
#31686=DIRECTION('center_axis',(0.,-1.,0.));
#31687=DIRECTION('ref_axis',(1.,0.,0.));
#31688=DIRECTION('',(0.,-1.,0.));
#31689=DIRECTION('center_axis',(0.,1.,0.));
#31690=DIRECTION('ref_axis',(1.,0.,0.));
#31691=DIRECTION('center_axis',(0.,1.,0.));
#31692=DIRECTION('ref_axis',(1.,0.,0.));
#31693=DIRECTION('center_axis',(0.,-1.,0.));
#31694=DIRECTION('ref_axis',(1.,0.,0.));
#31695=DIRECTION('',(-0.707106781186555,0.70710678118654,8.65956056235503E-17));
#31696=DIRECTION('center_axis',(0.,-1.,0.));
#31697=DIRECTION('ref_axis',(1.,0.,0.));
#31698=DIRECTION('',(0.,-1.,0.));
#31699=DIRECTION('center_axis',(0.,1.,0.));
#31700=DIRECTION('ref_axis',(1.,0.,0.));
#31701=DIRECTION('center_axis',(0.,1.,0.));
#31702=DIRECTION('ref_axis',(1.,0.,0.));
#31703=DIRECTION('center_axis',(0.,-1.,0.));
#31704=DIRECTION('ref_axis',(1.,0.,0.));
#31705=DIRECTION('',(-0.707106781186555,0.70710678118654,8.65956056235503E-17));
#31706=DIRECTION('center_axis',(0.,-1.,0.));
#31707=DIRECTION('ref_axis',(1.,0.,0.));
#31708=DIRECTION('',(0.,-1.,0.));
#31709=DIRECTION('center_axis',(0.,1.,0.));
#31710=DIRECTION('ref_axis',(1.,0.,0.));
#31711=DIRECTION('center_axis',(0.,1.,0.));
#31712=DIRECTION('ref_axis',(1.,0.,0.));
#31713=DIRECTION('center_axis',(0.,-1.,0.));
#31714=DIRECTION('ref_axis',(1.,0.,0.));
#31715=DIRECTION('',(-0.707106781186547,0.707106781186548,8.65956056235493E-17));
#31716=DIRECTION('center_axis',(0.,-1.,0.));
#31717=DIRECTION('ref_axis',(1.,0.,0.));
#31718=DIRECTION('',(0.,-1.,0.));
#31719=DIRECTION('center_axis',(0.,1.,0.));
#31720=DIRECTION('ref_axis',(1.,0.,0.));
#31721=DIRECTION('center_axis',(0.,1.,0.));
#31722=DIRECTION('ref_axis',(1.,0.,0.));
#31723=DIRECTION('center_axis',(0.,-1.,0.));
#31724=DIRECTION('ref_axis',(1.,0.,0.));
#31725=DIRECTION('',(-0.707106781186547,0.707106781186548,8.65956056235493E-17));
#31726=DIRECTION('center_axis',(0.,-1.,0.));
#31727=DIRECTION('ref_axis',(1.,0.,0.));
#31728=DIRECTION('',(0.,-1.,0.));
#31729=DIRECTION('center_axis',(0.,1.,0.));
#31730=DIRECTION('ref_axis',(1.,0.,0.));
#31731=DIRECTION('center_axis',(0.,1.,0.));
#31732=DIRECTION('ref_axis',(1.,0.,0.));
#31733=DIRECTION('center_axis',(0.,-1.,0.));
#31734=DIRECTION('ref_axis',(1.,0.,0.));
#31735=DIRECTION('',(-0.707106781186547,0.707106781186548,8.65956056235493E-17));
#31736=DIRECTION('center_axis',(0.,-1.,0.));
#31737=DIRECTION('ref_axis',(1.,0.,0.));
#31738=DIRECTION('',(0.,-1.,0.));
#31739=DIRECTION('center_axis',(0.,1.,0.));
#31740=DIRECTION('ref_axis',(1.,0.,0.));
#31741=DIRECTION('center_axis',(0.,1.,0.));
#31742=DIRECTION('ref_axis',(1.,0.,0.));
#31743=DIRECTION('center_axis',(0.,-1.,0.));
#31744=DIRECTION('ref_axis',(1.,0.,0.));
#31745=DIRECTION('',(-0.707106781186547,0.707106781186548,8.65956056235493E-17));
#31746=DIRECTION('center_axis',(0.,-1.,0.));
#31747=DIRECTION('ref_axis',(1.,0.,0.));
#31748=DIRECTION('',(0.,-1.,0.));
#31749=DIRECTION('center_axis',(0.,1.,0.));
#31750=DIRECTION('ref_axis',(1.,0.,0.));
#31751=DIRECTION('center_axis',(0.,1.,0.));
#31752=DIRECTION('ref_axis',(1.,0.,0.));
#31753=DIRECTION('center_axis',(0.,-1.,0.));
#31754=DIRECTION('ref_axis',(1.,0.,0.));
#31755=DIRECTION('',(-0.707106781186547,0.707106781186548,8.65956056235493E-17));
#31756=DIRECTION('center_axis',(0.,-1.,0.));
#31757=DIRECTION('ref_axis',(1.,0.,0.));
#31758=DIRECTION('',(0.,-1.,0.));
#31759=DIRECTION('center_axis',(0.,1.,0.));
#31760=DIRECTION('ref_axis',(1.,0.,0.));
#31761=DIRECTION('center_axis',(0.,1.,0.));
#31762=DIRECTION('ref_axis',(1.,0.,0.));
#31763=DIRECTION('center_axis',(0.,-1.,0.));
#31764=DIRECTION('ref_axis',(1.,0.,0.));
#31765=DIRECTION('',(-0.707106781186555,0.70710678118654,8.65956056235503E-17));
#31766=DIRECTION('center_axis',(0.,-1.,0.));
#31767=DIRECTION('ref_axis',(1.,0.,0.));
#31768=DIRECTION('',(0.,-1.,0.));
#31769=DIRECTION('center_axis',(0.,1.,0.));
#31770=DIRECTION('ref_axis',(1.,0.,0.));
#31771=DIRECTION('center_axis',(0.,1.,0.));
#31772=DIRECTION('ref_axis',(1.,0.,0.));
#31773=DIRECTION('center_axis',(0.,-1.,0.));
#31774=DIRECTION('ref_axis',(1.,0.,0.));
#31775=DIRECTION('',(-0.707106781186555,0.70710678118654,8.65956056235503E-17));
#31776=DIRECTION('center_axis',(0.,-1.,0.));
#31777=DIRECTION('ref_axis',(1.,0.,0.));
#31778=DIRECTION('',(0.,-1.,0.));
#31779=DIRECTION('center_axis',(0.,1.,0.));
#31780=DIRECTION('ref_axis',(1.,0.,0.));
#31781=DIRECTION('center_axis',(0.,1.,0.));
#31782=DIRECTION('ref_axis',(1.,0.,0.));
#31783=DIRECTION('center_axis',(0.,-1.,0.));
#31784=DIRECTION('ref_axis',(1.,0.,0.));
#31785=DIRECTION('',(-0.707106781186555,0.70710678118654,8.65956056235503E-17));
#31786=DIRECTION('center_axis',(0.,-1.,0.));
#31787=DIRECTION('ref_axis',(1.,0.,0.));
#31788=DIRECTION('',(0.,-1.,0.));
#31789=DIRECTION('center_axis',(0.,1.,0.));
#31790=DIRECTION('ref_axis',(1.,0.,0.));
#31791=DIRECTION('center_axis',(0.,1.,0.));
#31792=DIRECTION('ref_axis',(1.,0.,0.));
#31793=DIRECTION('center_axis',(0.,-1.,0.));
#31794=DIRECTION('ref_axis',(1.,0.,0.));
#31795=DIRECTION('',(-0.707106781186555,0.70710678118654,8.65956056235503E-17));
#31796=DIRECTION('center_axis',(0.,-1.,0.));
#31797=DIRECTION('ref_axis',(1.,0.,0.));
#31798=DIRECTION('',(0.,-1.,0.));
#31799=DIRECTION('center_axis',(0.,1.,0.));
#31800=DIRECTION('ref_axis',(1.,0.,0.));
#31801=DIRECTION('center_axis',(0.,1.,0.));
#31802=DIRECTION('ref_axis',(1.,0.,0.));
#31803=DIRECTION('center_axis',(0.,-1.,0.));
#31804=DIRECTION('ref_axis',(1.,0.,0.));
#31805=DIRECTION('',(-0.707106781186555,0.70710678118654,8.65956056235503E-17));
#31806=DIRECTION('center_axis',(0.,-1.,0.));
#31807=DIRECTION('ref_axis',(1.,0.,0.));
#31808=DIRECTION('',(0.,-1.,0.));
#31809=DIRECTION('center_axis',(0.,1.,0.));
#31810=DIRECTION('ref_axis',(1.,0.,0.));
#31811=DIRECTION('center_axis',(0.,1.,0.));
#31812=DIRECTION('ref_axis',(1.,0.,0.));
#31813=DIRECTION('center_axis',(0.,-1.,0.));
#31814=DIRECTION('ref_axis',(1.,0.,0.));
#31815=DIRECTION('',(-0.707106781186547,0.707106781186548,8.65956056235493E-17));
#31816=DIRECTION('center_axis',(0.,-1.,0.));
#31817=DIRECTION('ref_axis',(1.,0.,0.));
#31818=DIRECTION('',(0.,-1.,0.));
#31819=DIRECTION('center_axis',(0.,1.,0.));
#31820=DIRECTION('ref_axis',(1.,0.,0.));
#31821=DIRECTION('center_axis',(0.,1.,0.));
#31822=DIRECTION('ref_axis',(1.,0.,0.));
#31823=DIRECTION('center_axis',(0.,-1.,0.));
#31824=DIRECTION('ref_axis',(1.,0.,0.));
#31825=DIRECTION('',(-0.707106781186547,0.707106781186548,8.65956056235493E-17));
#31826=DIRECTION('center_axis',(0.,-1.,0.));
#31827=DIRECTION('ref_axis',(1.,0.,0.));
#31828=DIRECTION('',(0.,-1.,0.));
#31829=DIRECTION('center_axis',(0.,1.,0.));
#31830=DIRECTION('ref_axis',(1.,0.,0.));
#31831=DIRECTION('center_axis',(0.,1.,0.));
#31832=DIRECTION('ref_axis',(1.,0.,0.));
#31833=DIRECTION('center_axis',(0.,-1.,0.));
#31834=DIRECTION('ref_axis',(1.,0.,0.));
#31835=DIRECTION('',(-0.707106781186547,0.707106781186548,8.65956056235493E-17));
#31836=DIRECTION('center_axis',(0.,-1.,0.));
#31837=DIRECTION('ref_axis',(1.,0.,0.));
#31838=DIRECTION('',(0.,-1.,0.));
#31839=DIRECTION('center_axis',(0.,1.,0.));
#31840=DIRECTION('ref_axis',(1.,0.,0.));
#31841=DIRECTION('center_axis',(0.,0.707106781186541,0.707106781186554));
#31842=DIRECTION('ref_axis',(1.,0.,0.));
#31843=DIRECTION('',(0.,0.707106781186554,-0.707106781186541));
#31844=DIRECTION('',(0.,-0.707106781186554,0.707106781186541));
#31845=DIRECTION('',(1.,0.,0.));
#31846=DIRECTION('center_axis',(0.,-1.,0.));
#31847=DIRECTION('ref_axis',(0.,0.,1.));
#31848=DIRECTION('',(0.,0.707106781186547,0.707106781186547));
#31849=DIRECTION('center_axis',(0.,1.,0.));
#31850=DIRECTION('ref_axis',(0.,0.,1.));
#31851=DIRECTION('center_axis',(0.,0.707106781186543,-0.707106781186552));
#31852=DIRECTION('ref_axis',(-1.,0.,0.));
#31853=DIRECTION('',(0.,0.707106781186552,0.707106781186543));
#31854=DIRECTION('',(-1.,0.,0.));
#31855=DIRECTION('center_axis',(0.,-1.,0.));
#31856=DIRECTION('ref_axis',(0.,0.,-1.));
#31857=DIRECTION('center_axis',(0.,1.,0.));
#31858=DIRECTION('ref_axis',(0.,0.,-1.));
#31859=DIRECTION('center_axis',(0.,1.,0.));
#31860=DIRECTION('ref_axis',(0.,0.,1.));
#31861=DIRECTION('',(0.,1.,0.));
#31862=DIRECTION('center_axis',(0.,-1.,0.));
#31863=DIRECTION('ref_axis',(0.,0.,1.));
#31864=DIRECTION('',(0.,1.,0.));
#31865=DIRECTION('center_axis',(0.,0.,1.));
#31866=DIRECTION('ref_axis',(1.,0.,0.));
#31867=DIRECTION('',(0.,1.,0.));
#31868=DIRECTION('',(-1.,0.,0.));
#31869=DIRECTION('center_axis',(0.,-0.707106781186541,0.707106781186554));
#31870=DIRECTION('ref_axis',(1.,0.,0.));
#31871=DIRECTION('',(0.,-0.707106781186554,-0.707106781186541));
#31872=DIRECTION('',(1.,0.,0.));
#31873=DIRECTION('',(0.,0.707106781186554,0.707106781186541));
#31874=DIRECTION('center_axis',(0.,1.,0.));
#31875=DIRECTION('ref_axis',(0.,0.,-1.));
#31876=DIRECTION('center_axis',(0.,-1.,0.));
#31877=DIRECTION('ref_axis',(0.,0.,-1.));
#31878=DIRECTION('',(0.,-0.707106781186547,0.707106781186547));
#31879=DIRECTION('center_axis',(0.,1.,0.));
#31880=DIRECTION('ref_axis',(0.,0.,-1.));
#31881=DIRECTION('center_axis',(0.,-0.707106781186543,-0.707106781186552));
#31882=DIRECTION('ref_axis',(-1.,0.,0.));
#31883=DIRECTION('',(0.,-0.707106781186554,0.707106781186541));
#31884=DIRECTION('',(-1.,0.,0.));
#31885=DIRECTION('',(1.,0.,0.));
#31886=DIRECTION('center_axis',(0.,1.,0.));
#31887=DIRECTION('ref_axis',(0.,0.,1.));
#31888=DIRECTION('center_axis',(0.,1.,0.));
#31889=DIRECTION('ref_axis',(0.,0.,1.));
#31890=DIRECTION('center_axis',(0.,1.,0.));
#31891=DIRECTION('ref_axis',(0.,0.,-1.));
#31892=DIRECTION('',(0.,1.,0.));
#31893=DIRECTION('center_axis',(0.,1.,0.));
#31894=DIRECTION('ref_axis',(1.,0.,0.));
#31895=DIRECTION('center_axis',(0.,0.,-1.));
#31896=DIRECTION('ref_axis',(-1.,0.,0.));
#50671=CARTESIAN_POINT('',(0.,0.,0.));
#50672=CARTESIAN_POINT('Origin',(97.79,63.745,12.066));
#50673=CARTESIAN_POINT('',(96.012,63.645,12.066));
#50674=CARTESIAN_POINT('Origin',(97.79,63.645,12.066));
#50675=CARTESIAN_POINT('',(95.812,63.845,12.066));
#50676=CARTESIAN_POINT('',(95.912,63.745,12.066));
#50677=CARTESIAN_POINT('Origin',(97.79,63.845,12.066));
#50678=CARTESIAN_POINT('Origin',(0.,63.845,12.066));
#50679=CARTESIAN_POINT('',(97.79,63.845,16.5785));
#50680=CARTESIAN_POINT('',(-97.79,63.845,16.5785));
#50681=CARTESIAN_POINT('',(-48.895,63.845,16.5785));
#50682=CARTESIAN_POINT('',(97.79,63.845,7.5535));
#50683=CARTESIAN_POINT('Origin',(97.79,63.845,12.066));
#50684=CARTESIAN_POINT('',(-97.79,63.845,7.5535));
#50685=CARTESIAN_POINT('',(48.895,63.845,7.5535));
#50686=CARTESIAN_POINT('Origin',(-97.79,63.845,12.066));
#50687=CARTESIAN_POINT('',(76.254,63.845,12.066));
#50688=CARTESIAN_POINT('Origin',(78.232,63.845,12.066));
#50689=CARTESIAN_POINT('',(37.138,63.845,12.066));
#50690=CARTESIAN_POINT('Origin',(39.116,63.845,12.066));
#50691=CARTESIAN_POINT('',(-99.768,63.845,12.066));
#50692=CARTESIAN_POINT('Origin',(-97.79,63.845,12.066));
#50693=CARTESIAN_POINT('',(-31.315,63.845,12.066));
#50694=CARTESIAN_POINT('Origin',(-29.337,63.845,12.066));
#50695=CARTESIAN_POINT('',(-70.431,63.845,12.066));
#50696=CARTESIAN_POINT('Origin',(-68.453,63.845,12.066));
#50697=CARTESIAN_POINT('',(-80.21,63.845,12.066));
#50698=CARTESIAN_POINT('Origin',(-78.232,63.845,12.066));
#50699=CARTESIAN_POINT('',(-41.094,63.845,12.066));
#50700=CARTESIAN_POINT('Origin',(-39.116,63.845,12.066));
#50701=CARTESIAN_POINT('',(-1.978,63.845,12.066));
#50702=CARTESIAN_POINT('Origin',(0.,63.845,12.066));
#50703=CARTESIAN_POINT('',(27.359,63.845,12.066));
#50704=CARTESIAN_POINT('Origin',(29.337,63.845,12.066));
#50705=CARTESIAN_POINT('',(66.475,63.845,12.066));
#50706=CARTESIAN_POINT('Origin',(68.453,63.845,12.066));
#50707=CARTESIAN_POINT('',(86.033,63.845,12.066));
#50708=CARTESIAN_POINT('Origin',(88.011,63.845,12.066));
#50709=CARTESIAN_POINT('',(46.917,63.845,12.066));
#50710=CARTESIAN_POINT('Origin',(48.895,63.845,12.066));
#50711=CARTESIAN_POINT('',(7.801,63.845,12.066));
#50712=CARTESIAN_POINT('Origin',(9.779,63.845,12.066));
#50713=CARTESIAN_POINT('',(-21.536,63.845,12.066));
#50714=CARTESIAN_POINT('Origin',(-19.558,63.845,12.066));
#50715=CARTESIAN_POINT('',(-60.652,63.845,12.066));
#50716=CARTESIAN_POINT('Origin',(-58.674,63.845,12.066));
#50717=CARTESIAN_POINT('',(-89.989,63.845,12.066));
#50718=CARTESIAN_POINT('Origin',(-88.011,63.845,12.066));
#50719=CARTESIAN_POINT('',(-50.873,63.845,12.066));
#50720=CARTESIAN_POINT('Origin',(-48.895,63.845,12.066));
#50721=CARTESIAN_POINT('',(-11.757,63.845,12.066));
#50722=CARTESIAN_POINT('Origin',(-9.779,63.845,12.066));
#50723=CARTESIAN_POINT('',(17.58,63.845,12.066));
#50724=CARTESIAN_POINT('Origin',(19.558,63.845,12.066));
#50725=CARTESIAN_POINT('',(56.696,63.845,12.066));
#50726=CARTESIAN_POINT('Origin',(58.674,63.845,12.066));
#50727=CARTESIAN_POINT('Origin',(97.79,63.845,12.066));
#50728=CARTESIAN_POINT('',(96.012,57.495,12.066));
#50729=CARTESIAN_POINT('',(96.012,63.845,12.066));
#50730=CARTESIAN_POINT('Origin',(97.79,57.495,12.066));
#50731=CARTESIAN_POINT('Origin',(78.232,63.745,12.066));
#50732=CARTESIAN_POINT('',(76.454,63.645,12.066));
#50733=CARTESIAN_POINT('Origin',(78.232,63.645,12.066));
#50734=CARTESIAN_POINT('',(76.354,63.745,12.066));
#50735=CARTESIAN_POINT('Origin',(78.232,63.845,12.066));
#50736=CARTESIAN_POINT('',(76.454,57.495,12.066));
#50737=CARTESIAN_POINT('',(76.454,63.845,12.066));
#50738=CARTESIAN_POINT('Origin',(78.232,57.495,12.066));
#50739=CARTESIAN_POINT('Origin',(58.674,63.745,12.066));
#50740=CARTESIAN_POINT('',(56.896,63.645,12.066));
#50741=CARTESIAN_POINT('Origin',(58.674,63.645,12.066));
#50742=CARTESIAN_POINT('',(56.796,63.745,12.066));
#50743=CARTESIAN_POINT('Origin',(58.674,63.845,12.066));
#50744=CARTESIAN_POINT('',(56.896,57.495,12.066));
#50745=CARTESIAN_POINT('',(56.896,63.845,12.066));
#50746=CARTESIAN_POINT('Origin',(58.674,57.495,12.066));
#50747=CARTESIAN_POINT('Origin',(39.116,63.745,12.066));
#50748=CARTESIAN_POINT('',(37.338,63.645,12.066));
#50749=CARTESIAN_POINT('Origin',(39.116,63.645,12.066));
#50750=CARTESIAN_POINT('',(37.238,63.745,12.066));
#50751=CARTESIAN_POINT('Origin',(39.116,63.845,12.066));
#50752=CARTESIAN_POINT('',(37.338,57.495,12.066));
#50753=CARTESIAN_POINT('',(37.338,63.845,12.066));
#50754=CARTESIAN_POINT('Origin',(39.116,57.495,12.066));
#50755=CARTESIAN_POINT('Origin',(19.558,63.745,12.066));
#50756=CARTESIAN_POINT('',(17.78,63.645,12.066));
#50757=CARTESIAN_POINT('Origin',(19.558,63.645,12.066));
#50758=CARTESIAN_POINT('',(17.68,63.745,12.066));
#50759=CARTESIAN_POINT('Origin',(19.558,63.845,12.066));
#50760=CARTESIAN_POINT('',(17.78,57.495,12.066));
#50761=CARTESIAN_POINT('',(17.78,63.845,12.066));
#50762=CARTESIAN_POINT('Origin',(19.558,57.495,12.066));
#50763=CARTESIAN_POINT('Origin',(-97.79,63.745,12.066));
#50764=CARTESIAN_POINT('',(-99.568,63.645,12.066));
#50765=CARTESIAN_POINT('Origin',(-97.79,63.645,12.066));
#50766=CARTESIAN_POINT('',(-99.668,63.745,12.066));
#50767=CARTESIAN_POINT('Origin',(-97.79,63.845,12.066));
#50768=CARTESIAN_POINT('',(-99.568,57.495,12.066));
#50769=CARTESIAN_POINT('',(-99.568,63.845,12.066));
#50770=CARTESIAN_POINT('Origin',(-97.79,57.495,12.066));
#50771=CARTESIAN_POINT('Origin',(-9.779,63.745,12.066));
#50772=CARTESIAN_POINT('',(-11.557,63.645,12.066));
#50773=CARTESIAN_POINT('Origin',(-9.779,63.645,12.066));
#50774=CARTESIAN_POINT('',(-11.657,63.745,12.066));
#50775=CARTESIAN_POINT('Origin',(-9.779,63.845,12.066));
#50776=CARTESIAN_POINT('',(-11.557,57.495,12.066));
#50777=CARTESIAN_POINT('',(-11.557,63.845,12.066));
#50778=CARTESIAN_POINT('Origin',(-9.779,57.495,12.066));
#50779=CARTESIAN_POINT('Origin',(-29.337,63.745,12.066));
#50780=CARTESIAN_POINT('',(-31.115,63.645,12.066));
#50781=CARTESIAN_POINT('Origin',(-29.337,63.645,12.066));
#50782=CARTESIAN_POINT('',(-31.215,63.745,12.066));
#50783=CARTESIAN_POINT('Origin',(-29.337,63.845,12.066));
#50784=CARTESIAN_POINT('',(-31.115,57.495,12.066));
#50785=CARTESIAN_POINT('',(-31.115,63.845,12.066));
#50786=CARTESIAN_POINT('Origin',(-29.337,57.495,12.066));
#50787=CARTESIAN_POINT('Origin',(-48.895,63.745,12.066));
#50788=CARTESIAN_POINT('',(-50.673,63.645,12.066));
#50789=CARTESIAN_POINT('Origin',(-48.895,63.645,12.066));
#50790=CARTESIAN_POINT('',(-50.773,63.745,12.066));
#50791=CARTESIAN_POINT('Origin',(-48.895,63.845,12.066));
#50792=CARTESIAN_POINT('',(-50.673,57.495,12.066));
#50793=CARTESIAN_POINT('',(-50.673,63.845,12.066));
#50794=CARTESIAN_POINT('Origin',(-48.895,57.495,12.066));
#50795=CARTESIAN_POINT('Origin',(-68.453,63.745,12.066));
#50796=CARTESIAN_POINT('',(-70.231,63.645,12.066));
#50797=CARTESIAN_POINT('Origin',(-68.453,63.645,12.066));
#50798=CARTESIAN_POINT('',(-70.331,63.745,12.066));
#50799=CARTESIAN_POINT('Origin',(-68.453,63.845,12.066));
#50800=CARTESIAN_POINT('',(-70.231,57.495,12.066));
#50801=CARTESIAN_POINT('',(-70.231,63.845,12.066));
#50802=CARTESIAN_POINT('Origin',(-68.453,57.495,12.066));
#50803=CARTESIAN_POINT('Origin',(-88.011,63.745,12.066));
#50804=CARTESIAN_POINT('',(-89.789,63.645,12.066));
#50805=CARTESIAN_POINT('Origin',(-88.011,63.645,12.066));
#50806=CARTESIAN_POINT('',(-89.889,63.745,12.066));
#50807=CARTESIAN_POINT('Origin',(-88.011,63.845,12.066));
#50808=CARTESIAN_POINT('',(-89.789,57.495,12.066));
#50809=CARTESIAN_POINT('',(-89.789,63.845,12.066));
#50810=CARTESIAN_POINT('Origin',(-88.011,57.495,12.066));
#50811=CARTESIAN_POINT('Origin',(-78.232,63.745,12.066));
#50812=CARTESIAN_POINT('',(-80.01,63.645,12.066));
#50813=CARTESIAN_POINT('Origin',(-78.232,63.645,12.066));
#50814=CARTESIAN_POINT('',(-80.11,63.745,12.066));
#50815=CARTESIAN_POINT('Origin',(-78.232,63.845,12.066));
#50816=CARTESIAN_POINT('',(-80.01,57.495,12.066));
#50817=CARTESIAN_POINT('',(-80.01,63.845,12.066));
#50818=CARTESIAN_POINT('Origin',(-78.232,57.495,12.066));
#50819=CARTESIAN_POINT('Origin',(-58.674,63.745,12.066));
#50820=CARTESIAN_POINT('',(-60.452,63.645,12.066));
#50821=CARTESIAN_POINT('Origin',(-58.674,63.645,12.066));
#50822=CARTESIAN_POINT('',(-60.552,63.745,12.066));
#50823=CARTESIAN_POINT('Origin',(-58.674,63.845,12.066));
#50824=CARTESIAN_POINT('',(-60.452,57.495,12.066));
#50825=CARTESIAN_POINT('',(-60.452,63.845,12.066));
#50826=CARTESIAN_POINT('Origin',(-58.674,57.495,12.066));
#50827=CARTESIAN_POINT('Origin',(-39.116,63.745,12.066));
#50828=CARTESIAN_POINT('',(-40.894,63.645,12.066));
#50829=CARTESIAN_POINT('Origin',(-39.116,63.645,12.066));
#50830=CARTESIAN_POINT('',(-40.994,63.745,12.066));
#50831=CARTESIAN_POINT('Origin',(-39.116,63.845,12.066));
#50832=CARTESIAN_POINT('',(-40.894,57.495,12.066));
#50833=CARTESIAN_POINT('',(-40.894,63.845,12.066));
#50834=CARTESIAN_POINT('Origin',(-39.116,57.495,12.066));
#50835=CARTESIAN_POINT('Origin',(-19.558,63.745,12.066));
#50836=CARTESIAN_POINT('',(-21.336,63.645,12.066));
#50837=CARTESIAN_POINT('Origin',(-19.558,63.645,12.066));
#50838=CARTESIAN_POINT('',(-21.436,63.745,12.066));
#50839=CARTESIAN_POINT('Origin',(-19.558,63.845,12.066));
#50840=CARTESIAN_POINT('',(-21.336,57.495,12.066));
#50841=CARTESIAN_POINT('',(-21.336,63.845,12.066));
#50842=CARTESIAN_POINT('Origin',(-19.558,57.495,12.066));
#50843=CARTESIAN_POINT('Origin',(0.,63.745,12.066));
#50844=CARTESIAN_POINT('',(-1.778,63.645,12.066));
#50845=CARTESIAN_POINT('Origin',(0.,63.645,12.066));
#50846=CARTESIAN_POINT('',(-1.878,63.745,12.066));
#50847=CARTESIAN_POINT('Origin',(0.,63.845,12.066));
#50848=CARTESIAN_POINT('',(-1.778,57.495,12.066));
#50849=CARTESIAN_POINT('',(-1.778,63.845,12.066));
#50850=CARTESIAN_POINT('Origin',(0.,57.495,12.066));
#50851=CARTESIAN_POINT('Origin',(9.779,63.745,12.066));
#50852=CARTESIAN_POINT('',(8.001,63.645,12.066));
#50853=CARTESIAN_POINT('Origin',(9.779,63.645,12.066));
#50854=CARTESIAN_POINT('',(7.901,63.745,12.066));
#50855=CARTESIAN_POINT('Origin',(9.779,63.845,12.066));
#50856=CARTESIAN_POINT('',(8.001,57.495,12.066));
#50857=CARTESIAN_POINT('',(8.001,63.845,12.066));
#50858=CARTESIAN_POINT('Origin',(9.779,57.495,12.066));
#50859=CARTESIAN_POINT('Origin',(29.337,63.745,12.066));
#50860=CARTESIAN_POINT('',(27.559,63.645,12.066));
#50861=CARTESIAN_POINT('Origin',(29.337,63.645,12.066));
#50862=CARTESIAN_POINT('',(27.459,63.745,12.066));
#50863=CARTESIAN_POINT('Origin',(29.337,63.845,12.066));
#50864=CARTESIAN_POINT('',(27.559,57.495,12.066));
#50865=CARTESIAN_POINT('',(27.559,63.845,12.066));
#50866=CARTESIAN_POINT('Origin',(29.337,57.495,12.066));
#50867=CARTESIAN_POINT('Origin',(48.895,63.745,12.066));
#50868=CARTESIAN_POINT('',(47.117,63.645,12.066));
#50869=CARTESIAN_POINT('Origin',(48.895,63.645,12.066));
#50870=CARTESIAN_POINT('',(47.017,63.745,12.066));
#50871=CARTESIAN_POINT('Origin',(48.895,63.845,12.066));
#50872=CARTESIAN_POINT('',(47.117,57.495,12.066));
#50873=CARTESIAN_POINT('',(47.117,63.845,12.066));
#50874=CARTESIAN_POINT('Origin',(48.895,57.495,12.066));
#50875=CARTESIAN_POINT('Origin',(68.453,63.745,12.066));
#50876=CARTESIAN_POINT('',(66.675,63.645,12.066));
#50877=CARTESIAN_POINT('Origin',(68.453,63.645,12.066));
#50878=CARTESIAN_POINT('',(66.575,63.745,12.066));
#50879=CARTESIAN_POINT('Origin',(68.453,63.845,12.066));
#50880=CARTESIAN_POINT('',(66.675,57.495,12.066));
#50881=CARTESIAN_POINT('',(66.675,63.845,12.066));
#50882=CARTESIAN_POINT('Origin',(68.453,57.495,12.066));
#50883=CARTESIAN_POINT('Origin',(88.011,63.745,12.066));
#50884=CARTESIAN_POINT('',(86.233,63.645,12.066));
#50885=CARTESIAN_POINT('Origin',(88.011,63.645,12.066));
#50886=CARTESIAN_POINT('',(86.133,63.745,12.066));
#50887=CARTESIAN_POINT('Origin',(88.011,63.845,12.066));
#50888=CARTESIAN_POINT('',(86.233,57.495,12.066));
#50889=CARTESIAN_POINT('',(86.233,63.845,12.066));
#50890=CARTESIAN_POINT('Origin',(88.011,57.495,12.066));
#50891=CARTESIAN_POINT('Origin',(-48.895,63.72,16.7035));
#50892=CARTESIAN_POINT('',(97.79,63.595,16.8285));
#50893=CARTESIAN_POINT('',(97.79,63.595,16.8285));
#50894=CARTESIAN_POINT('',(-97.79,63.595,16.8285));
#50895=CARTESIAN_POINT('',(-97.79,63.845,16.5785));
#50896=CARTESIAN_POINT('',(-48.895,63.595,16.8285));
#50897=CARTESIAN_POINT('Origin',(97.79,63.72,12.066));
#50898=CARTESIAN_POINT('',(97.79,63.595,7.3035));
#50899=CARTESIAN_POINT('',(97.79,63.595,7.3035));
#50900=CARTESIAN_POINT('Origin',(97.79,63.595,12.066));
#50901=CARTESIAN_POINT('Origin',(48.895,63.72,7.4285));
#50902=CARTESIAN_POINT('',(-97.79,63.595,7.3035));
#50903=CARTESIAN_POINT('',(-97.79,63.595,7.3035));
#50904=CARTESIAN_POINT('',(48.895,63.595,7.3035));
#50905=CARTESIAN_POINT('Origin',(-97.79,63.72,12.066));
#50906=CARTESIAN_POINT('Origin',(-97.79,63.595,12.066));
#50907=CARTESIAN_POINT('Origin',(97.79,57.495,12.066));
#50908=CARTESIAN_POINT('',(97.79,57.745,16.8285));
#50909=CARTESIAN_POINT('',(97.79,57.495,16.8285));
#50910=CARTESIAN_POINT('',(97.79,57.745,7.3035));
#50911=CARTESIAN_POINT('Origin',(97.79,57.745,12.066));
#50912=CARTESIAN_POINT('',(97.79,57.495,7.3035));
#50913=CARTESIAN_POINT('Origin',(-97.79,57.495,16.8285));
#50914=CARTESIAN_POINT('',(-97.79,57.745,16.8285));
#50915=CARTESIAN_POINT('',(-97.79,57.495,16.8285));
#50916=CARTESIAN_POINT('',(-48.895,57.745,16.8285));
#50917=CARTESIAN_POINT('Origin',(-48.895,57.62,16.7035));
#50918=CARTESIAN_POINT('',(-97.79,57.495,16.5785));
#50919=CARTESIAN_POINT('',(-97.79,57.745,16.8285));
#50920=CARTESIAN_POINT('',(97.79,57.495,16.5785));
#50921=CARTESIAN_POINT('',(-48.895,57.495,16.5785));
#50922=CARTESIAN_POINT('',(97.79,57.495,16.5785));
#50923=CARTESIAN_POINT('Origin',(-97.79,57.62,12.066));
#50924=CARTESIAN_POINT('',(-97.79,57.745,7.3035));
#50925=CARTESIAN_POINT('Origin',(-97.79,57.745,12.066));
#50926=CARTESIAN_POINT('',(-97.79,57.495,7.5535));
#50927=CARTESIAN_POINT('',(-97.79,57.745,7.3035));
#50928=CARTESIAN_POINT('Origin',(-97.79,57.495,12.066));
#50929=CARTESIAN_POINT('Origin',(48.895,57.62,7.4285));
#50930=CARTESIAN_POINT('',(97.79,57.495,7.5535));
#50931=CARTESIAN_POINT('',(97.79,57.745,7.3035));
#50932=CARTESIAN_POINT('',(48.895,57.495,7.5535));
#50933=CARTESIAN_POINT('',(48.895,57.745,7.3035));
#50934=CARTESIAN_POINT('Origin',(97.79,57.62,12.066));
#50935=CARTESIAN_POINT('Origin',(97.79,57.495,12.066));
#50936=CARTESIAN_POINT('Origin',(-97.79,57.495,12.066));
#50937=CARTESIAN_POINT('',(-97.79,57.495,7.3035));
#50938=CARTESIAN_POINT('Origin',(0.,57.495,12.066));
#50939=CARTESIAN_POINT('Origin',(97.79,57.495,7.3035));
#83194=UNCERTAINTY_MEASURE_WITH_UNIT(LENGTH_MEASURE(0.01),#83220,
'DISTANCE_ACCURACY_VALUE',
'Maximum model space distance between geometric entities at asserted c
onnectivities');
#83203=UNCERTAINTY_MEASURE_WITH_UNIT(LENGTH_MEASURE(0.01),#83220,
'DISTANCE_ACCURACY_VALUE',
'Maximum model space distance between geometric entities at asserted c
onnectivities');
#83210=(
GEOMETRIC_REPRESENTATION_CONTEXT(3)
GLOBAL_UNCERTAINTY_ASSIGNED_CONTEXT((#83194))
GLOBAL_UNIT_ASSIGNED_CONTEXT((#83220,#83222,#83223))
REPRESENTATION_CONTEXT('','3D')
);
#83219=(
GEOMETRIC_REPRESENTATION_CONTEXT(3)
GLOBAL_UNCERTAINTY_ASSIGNED_CONTEXT((#83203))
GLOBAL_UNIT_ASSIGNED_CONTEXT((#83220,#83222,#83223))
REPRESENTATION_CONTEXT('','3D')
);
#83220=(
LENGTH_UNIT()
NAMED_UNIT(*)
SI_UNIT(.MILLI.,.METRE.)
);
#83222=(
NAMED_UNIT(*)
PLANE_ANGLE_UNIT()
SI_UNIT($,.RADIAN.)
);
#83223=(
NAMED_UNIT(*)
SI_UNIT($,.STERADIAN.)
SOLID_ANGLE_UNIT()
);
#83230=SHAPE_DEFINITION_REPRESENTATION(#83245,#83305);
#83245=PRODUCT_DEFINITION_SHAPE('',$,#83321);
#83305=SHAPE_REPRESENTATION('',(#27872),#83210);
#83314=PRODUCT_DEFINITION_CONTEXT('part definition',#83361,'design');
#83321=PRODUCT_DEFINITION('Aluminum Beam (cut to 21 holes)',
'Aluminum Beam (cut to 21 holes)',#83336,#83314);
#83336=PRODUCT_DEFINITION_FORMATION('',$,#83369);
#83361=APPLICATION_CONTEXT(
'Core Data for Automotive Mechanical Design Process');
#83362=PRODUCT_CONTEXT('part definition',#83361,'mechanical');
#83369=PRODUCT('Aluminum Beam (cut to 21 holes)',
'Aluminum Beam (cut to 21 holes)',$,(#83362));
#83384=PRESENTATION_STYLE_ASSIGNMENT((#83399));
#83399=SURFACE_STYLE_USAGE(.BOTH.,#83414);
#83414=SURFACE_SIDE_STYLE('',(#83429));
#83429=SURFACE_STYLE_FILL_AREA(#83444);
#83444=FILL_AREA_STYLE('Opaque(228,231,235)',(#83459));
#83459=FILL_AREA_STYLE_COLOUR('Opaque(228,231,235)',#83474);
#83474=COLOUR_RGB('Opaque(228,231,235)', 0.09019608, 0.27058824, 0.51372549);
ENDSEC;
END-ISO-10303-21;
